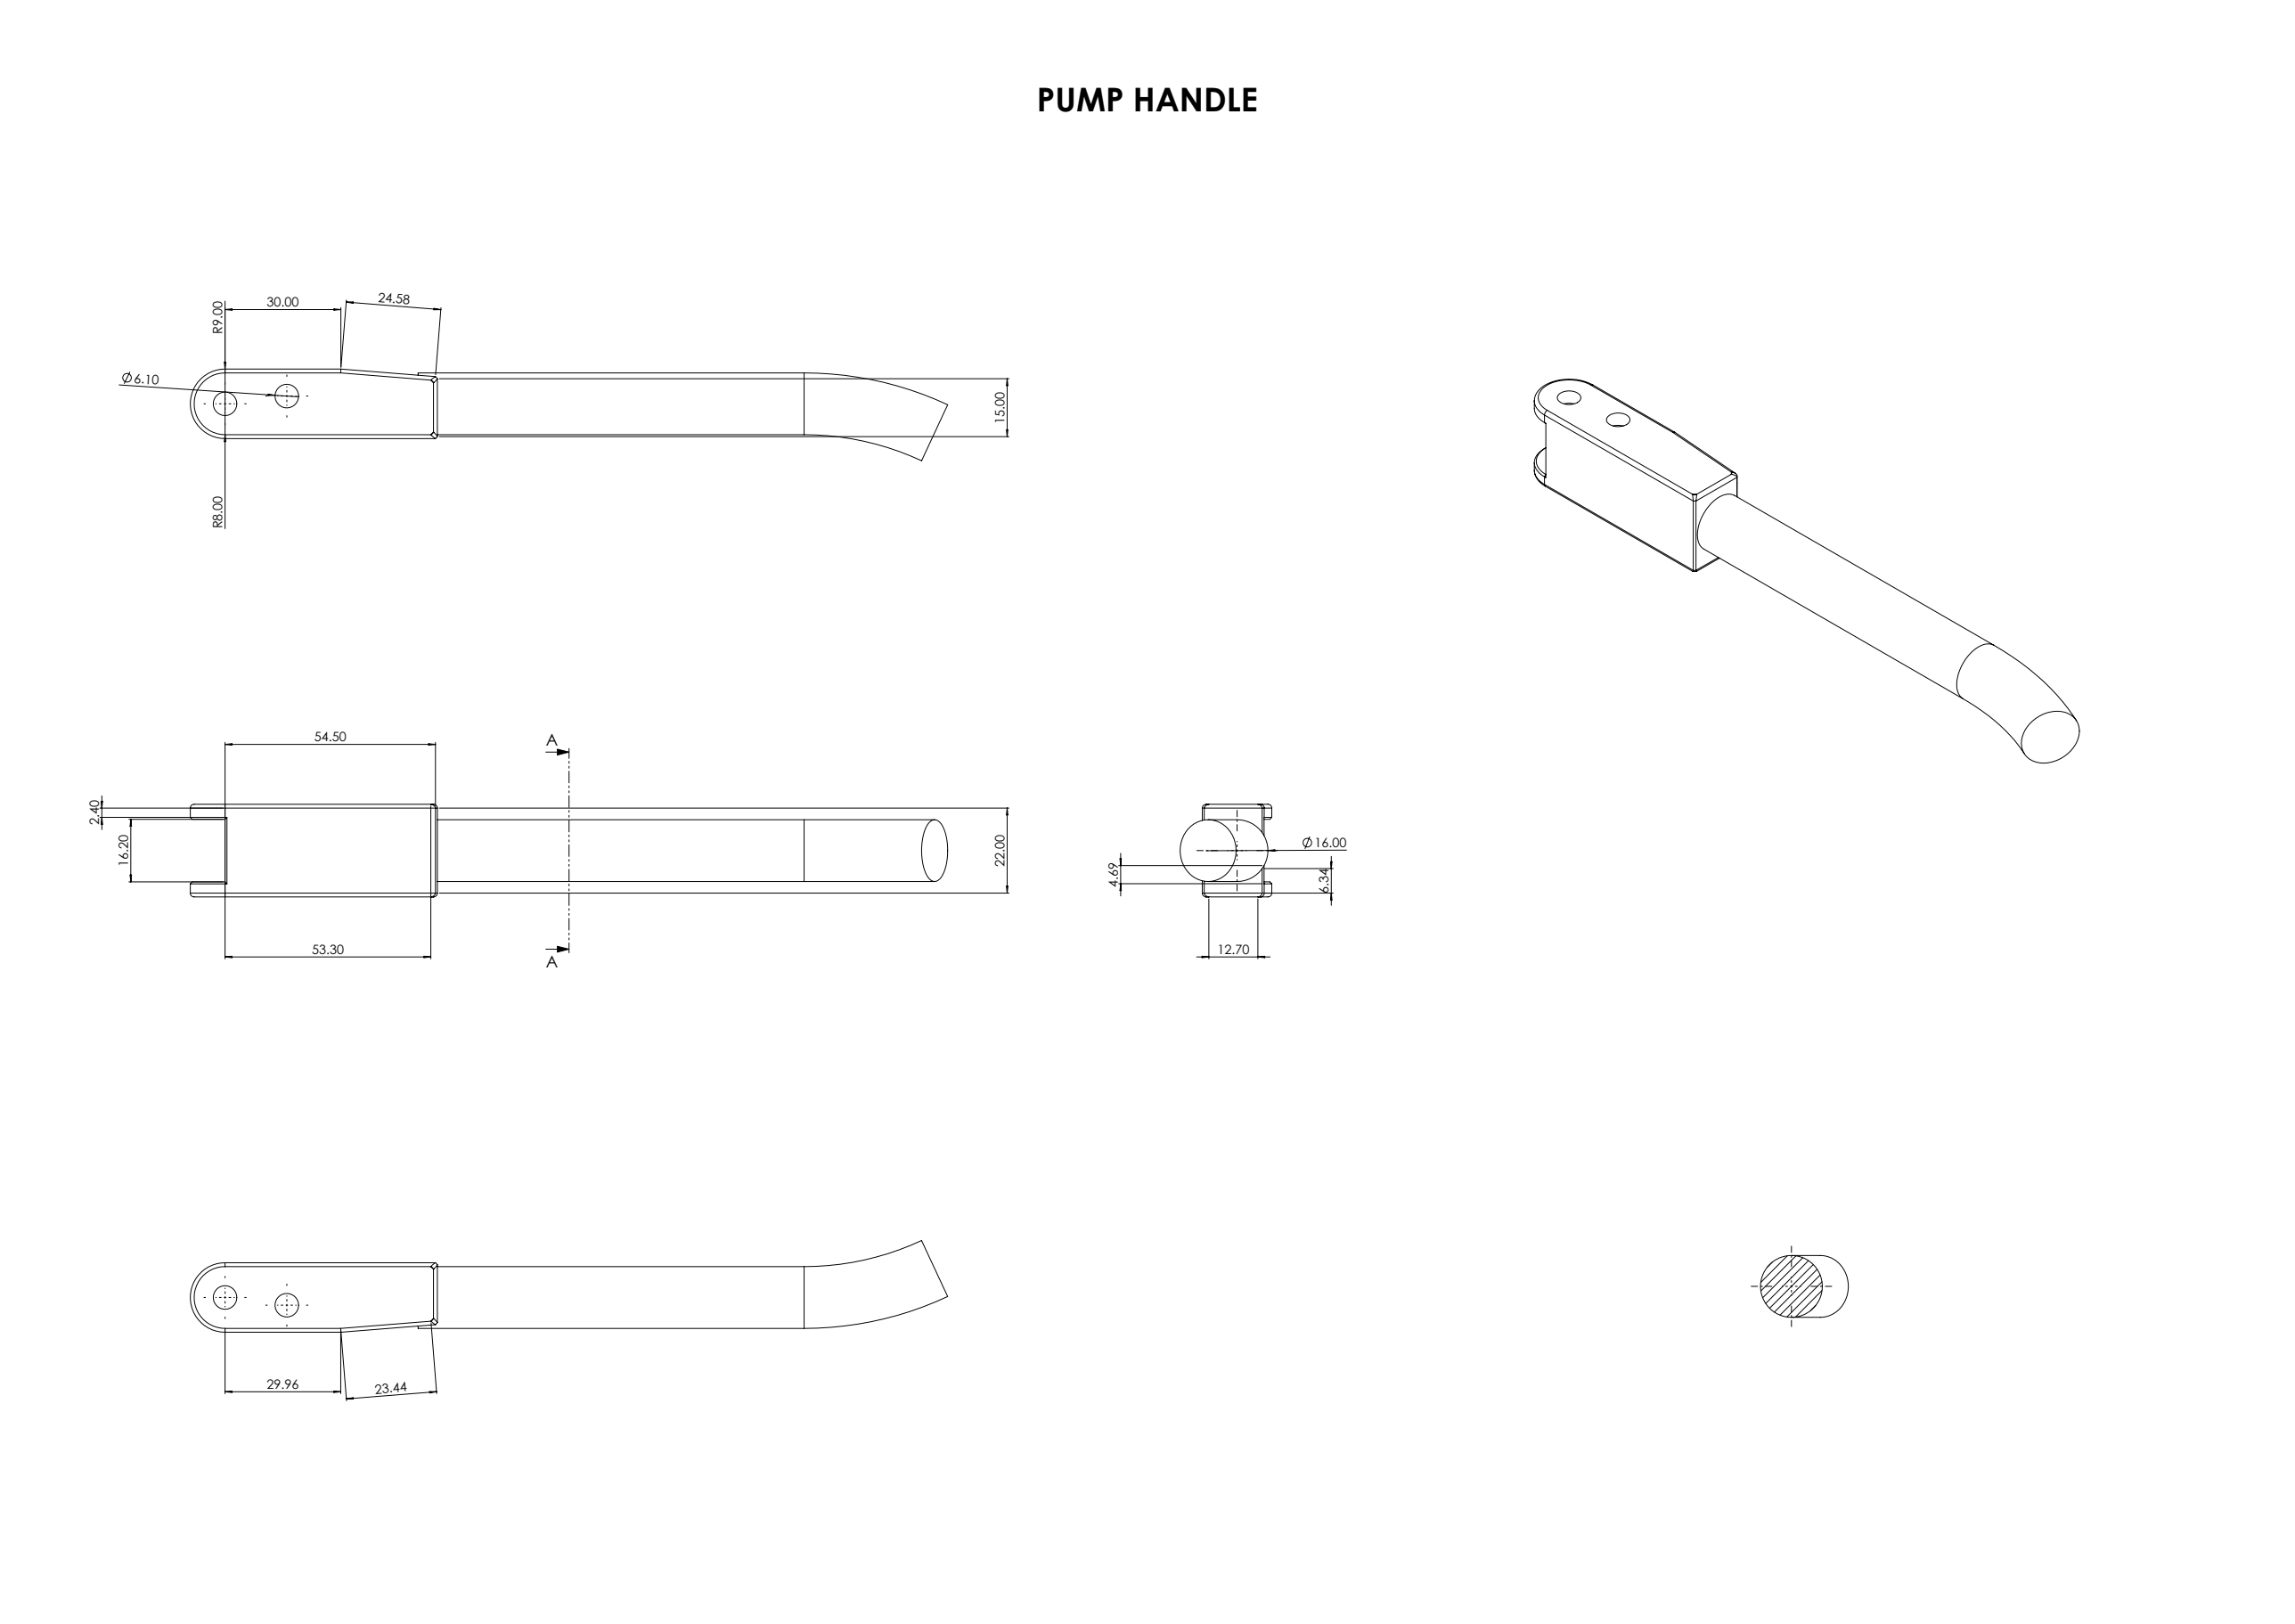
ISO-10303-21;
HEADER;
/* Generated by software containing ST-Developer
 * from STEP Tools, Inc. (www.steptools.com) 
 */

FILE_DESCRIPTION(
/* description */ (''),
/* implementation_level */ '2;1');

FILE_NAME(
/* name */ '14_Pump_Handle.step',
/* time_stamp */ '2026-10-26T03:55:20-07:00',
/* author */ (''),
/* organization */ (''),
/* preprocessor_version */ 'ST-DEVELOPER v20.2',
/* originating_system */ 'Autodesk Translation Framework v15.15.0.0',
/* authorisation */ '');

FILE_SCHEMA (('AUTOMOTIVE_DESIGN { 1 0 10303 214 3 1 1 }'));
ENDSEC;

DATA;
#10=MECHANICAL_DESIGN_GEOMETRIC_PRESENTATION_REPRESENTATION('',(#189),#45236);
#149=SHAPE_REPRESENTATION_RELATIONSHIP('SRR','None',#45328,#169);
#169=ADVANCED_BREP_SHAPE_REPRESENTATION('',(#209),#45230);
#189=STYLED_ITEM('',(#45498),#209);
#209=MANIFOLD_SOLID_BREP('Body1',#16531);
#225=TOROIDAL_SURFACE('',#17931,8.,1.);
#226=TOROIDAL_SURFACE('',#17938,8.,1.);
#227=TOROIDAL_SURFACE('',#17951,79.9999999999995,8.);
#252=ELLIPSE('',#17900,10.8879054120476,8.);
#253=ELLIPSE('',#17908,10.8879054120476,8.);
#254=ELLIPSE('',#17918,1.00079713248425,1.);
#255=ELLIPSE('',#17937,1.00079713248425,1.);
#790=B_SPLINE_CURVE_WITH_KNOTS('',3,(#44019,#44020,#44021,#44022,#44023,
#44024,#44025,#44026,#44027,#44028,#44029,#44030,#44031,#44032,#44033,#44034,
#44035,#44036,#44037,#44038,#44039,#44040,#44041,#44042,#44043,#44044,#44045,
#44046,#44047,#44048,#44049,#44050,#44051,#44052,#44053,#44054,#44055,#44056,
#44057,#44058,#44059,#44060,#44061,#44062,#44063,#44064,#44065,#44066,#44067,
#44068,#44069,#44070,#44071,#44072,#44073),.UNSPECIFIED.,.F.,.F.,(4,3,3,
3,3,3,3,3,3,3,3,3,3,3,3,3,3,3,4),(0.,0.0457286896420428,0.093735766404543,
0.144908104483403,0.201496379478659,0.273083254680907,0.346956864852629,
0.403665327235726,0.454892838429364,0.50491934325277,0.554438098871657,
0.607768246203659,0.669007112544933,0.7517553344087,0.813816500806525,0.866510270075527,
0.916070793074055,0.962308549660881,1.),.UNSPECIFIED.);
#791=B_SPLINE_CURVE_WITH_KNOTS('',3,(#44075,#44076,#44077,#44078),
 .UNSPECIFIED.,.F.,.F.,(4,4),(0.,1.),.UNSPECIFIED.);
#792=B_SPLINE_CURVE_WITH_KNOTS('',3,(#44080,#44081,#44082,#44083,#44084,
#44085,#44086,#44087,#44088,#44089,#44090,#44091,#44092,#44093,#44094,#44095,
#44096,#44097,#44098,#44099,#44100,#44101,#44102,#44103,#44104,#44105,#44106,
#44107,#44108,#44109,#44110,#44111,#44112,#44113,#44114,#44115,#44116,#44117,
#44118,#44119,#44120,#44121,#44122,#44123,#44124,#44125,#44126,#44127,#44128,
#44129,#44130,#44131,#44132,#44133,#44134),.UNSPECIFIED.,.F.,.F.,(4,3,3,
3,3,3,3,3,3,3,3,3,3,3,3,3,3,3,4),(0.,0.0457354346940703,0.0937501435458722,
0.144931624161072,0.20153359300957,0.273162634682721,0.347001992162202,
0.403710204556331,0.454939815804421,0.505015264674136,0.55453467353116,
0.607869111005662,0.669124504105853,0.75184337807939,0.813882533559542,
0.866563287605176,0.916113481178306,0.962343356347582,1.),.UNSPECIFIED.);
#793=B_SPLINE_CURVE_WITH_KNOTS('',3,(#44161,#44162,#44163,#44164,#44165,
#44166),.UNSPECIFIED.,.F.,.F.,(4,1,1,4),(-1.83137755752329,-1.04650146144188,
-0.52325073072094,-1.12036785251785E-15),.UNSPECIFIED.);
#794=B_SPLINE_CURVE_WITH_KNOTS('',3,(#44169,#44170,#44171,#44172,#44173,
#44174),.UNSPECIFIED.,.F.,.F.,(4,1,1,4),(1.12036785251785E-15,0.52325073072094,
1.04650146144188,1.83137755752329),.UNSPECIFIED.);
#795=B_SPLINE_CURVE_WITH_KNOTS('',3,(#44202,#44203,#44204,#44205,#44206,
#44207,#44208),.UNSPECIFIED.,.F.,.F.,(4,1,1,1,4),(-1.84798528578773,-1.0559915918787,
-0.527995795939349,-0.263997897969673,2.22044604925035E-15),
 .UNSPECIFIED.);
#796=B_SPLINE_CURVE_WITH_KNOTS('',3,(#44209,#44210,#44211,#44212,#44213,
#44214,#44215,#44216,#44217,#44218,#44219,#44220,#44221,#44222,#44223,#44224,
#44225,#44226,#44227,#44228,#44229,#44230,#44231,#44232,#44233,#44234,#44235,
#44236,#44237,#44238,#44239,#44240,#44241,#44242,#44243,#44244,#44245,#44246,
#44247,#44248,#44249,#44250,#44251,#44252,#44253,#44254,#44255,#44256,#44257,
#44258,#44259,#44260,#44261,#44262,#44263),.UNSPECIFIED.,.F.,.F.,(4,3,3,
3,3,3,3,3,3,3,3,3,3,3,3,3,3,3,4),(0.,0.0457132863749496,0.0937034140726246,
0.144856244328766,0.201417245857591,0.272937663581204,0.346860860114579,
0.403562222955401,0.454780120675855,0.503694405033869,0.553118113908822,
0.606292311523956,0.667190059273958,0.750392544455468,0.812794408341601,
0.865541001719504,0.91513380035021,0.961377819679936,1.),.UNSPECIFIED.);
#797=B_SPLINE_CURVE_WITH_KNOTS('',3,(#44305,#44306,#44307,#44308,#44309,
#44310,#44311,#44312,#44313,#44314,#44315,#44316,#44317,#44318,#44319,#44320,
#44321,#44322,#44323,#44324,#44325,#44326,#44327,#44328,#44329,#44330,#44331,
#44332,#44333,#44334,#44335,#44336,#44337,#44338,#44339,#44340,#44341,#44342,
#44343,#44344,#44345,#44346,#44347,#44348,#44349,#44350,#44351,#44352,#44353,
#44354,#44355,#44356,#44357,#44358,#44359),.UNSPECIFIED.,.F.,.F.,(4,3,3,
3,3,3,3,3,3,3,3,3,3,3,3,3,3,3,4),(0.,0.0457286896420497,0.0937357664051448,
0.144908104483507,0.201496379477572,0.273083254679073,0.34695686485381,
0.403665327236825,0.454892838430446,0.504919343256333,0.554438098874351,
0.607768246204756,0.669007112545538,0.751755334409154,0.813816500806865,
0.866510270075756,0.916070793073951,0.962308549660669,1.),.UNSPECIFIED.);
#798=B_SPLINE_CURVE_WITH_KNOTS('',3,(#44361,#44362,#44363,#44364),
 .UNSPECIFIED.,.F.,.F.,(4,4),(0.,1.),.UNSPECIFIED.);
#799=B_SPLINE_CURVE_WITH_KNOTS('',3,(#44366,#44367,#44368,#44369,#44370,
#44371,#44372,#44373,#44374,#44375,#44376,#44377,#44378,#44379,#44380,#44381,
#44382,#44383,#44384,#44385,#44386,#44387,#44388,#44389,#44390,#44391,#44392,
#44393,#44394,#44395,#44396,#44397,#44398,#44399,#44400,#44401,#44402,#44403,
#44404,#44405,#44406,#44407,#44408,#44409,#44410,#44411,#44412,#44413,#44414,
#44415,#44416,#44417,#44418,#44419,#44420),.UNSPECIFIED.,.F.,.F.,(4,3,3,
3,3,3,3,3,3,3,3,3,3,3,3,3,3,3,4),(0.,0.0457354346944535,0.0937501435463771,
0.144931624161605,0.201533593009091,0.273162634682324,0.347001992161254,
0.40371020455566,0.454939815803727,0.505015264672052,0.554534673528658,
0.607869111002009,0.669124504101831,0.751843378076374,0.81388253355728,
0.866563287602945,0.916113481176235,0.962343356345523,1.),.UNSPECIFIED.);
#800=B_SPLINE_CURVE_WITH_KNOTS('',3,(#44446,#44447,#44448,#44449,#44450,
#44451),.UNSPECIFIED.,.F.,.F.,(4,1,1,4),(-1.83137755752328,-1.04650146144188,
-0.523250730720938,-1.19348975147204E-15),.UNSPECIFIED.);
#801=B_SPLINE_CURVE_WITH_KNOTS('',3,(#44452,#44453,#44454,#44455,#44456,
#44457),.UNSPECIFIED.,.F.,.F.,(4,1,1,4),(1.19348975147204E-15,0.523250730720938,
1.04650146144188,1.83137755752328),.UNSPECIFIED.);
#802=B_SPLINE_CURVE_WITH_KNOTS('',3,(#44508,#44509,#44510,#44511),
 .UNSPECIFIED.,.F.,.F.,(4,4),(0.,1.),.UNSPECIFIED.);
#803=B_SPLINE_CURVE_WITH_KNOTS('',3,(#44512,#44513,#44514,#44515,#44516,
#44517,#44518,#44519,#44520,#44521,#44522,#44523,#44524,#44525,#44526,#44527,
#44528,#44529,#44530,#44531,#44532,#44533,#44534,#44535,#44536,#44537,#44538,
#44539,#44540,#44541,#44542,#44543,#44544,#44545,#44546,#44547,#44548,#44549,
#44550,#44551,#44552,#44553,#44554,#44555,#44556,#44557,#44558,#44559,#44560,
#44561,#44562,#44563,#44564,#44565,#44566),.UNSPECIFIED.,.F.,.F.,(4,3,3,
3,3,3,3,3,3,3,3,3,3,3,3,3,3,3,4),(0.,0.0457192684189794,0.0937161650457905,
0.144877103812885,0.201450247057813,0.273008005410247,0.346900713129524,
0.403601873101028,0.454821643624999,0.503755854254589,0.553178607570083,
0.606353906221449,0.667259789018953,0.750444841764215,0.812833631323161,
0.865569987859207,0.915154528460697,0.961391964978838,1.),.UNSPECIFIED.);
#804=B_SPLINE_CURVE_WITH_KNOTS('',3,(#44601,#44602,#44603,#44604,#44605,
#44606,#44607,#44608,#44609,#44610,#44611,#44612,#44613,#44614,#44615,#44616,
#44617,#44618,#44619,#44620,#44621,#44622,#44623,#44624,#44625,#44626,#44627,
#44628,#44629,#44630,#44631,#44632,#44633,#44634,#44635,#44636,#44637,#44638,
#44639,#44640,#44641,#44642,#44643,#44644,#44645,#44646,#44647,#44648,#44649,
#44650,#44651,#44652,#44653,#44654,#44655),.UNSPECIFIED.,.F.,.F.,(4,3,3,
3,3,3,3,3,3,3,3,3,3,3,3,3,3,3,4),(0.,0.0457132863751776,0.093703414073713,
0.144856244329965,0.201417245862007,0.272937663588709,0.346860860113243,
0.403562222954799,0.454780120675612,0.503694405126385,0.553118114005435,
0.60629231162977,0.667190059400792,0.750392544550594,0.812794408412946,
0.865541001786358,0.915133800413365,0.961377819741294,1.),.UNSPECIFIED.);
#805=B_SPLINE_CURVE_WITH_KNOTS('',3,(#44657,#44658,#44659,#44660),
 .UNSPECIFIED.,.F.,.F.,(4,4),(0.,1.),.UNSPECIFIED.);
#806=B_SPLINE_CURVE_WITH_KNOTS('',3,(#44662,#44663,#44664,#44665,#44666,
#44667,#44668,#44669,#44670,#44671,#44672,#44673,#44674,#44675,#44676,#44677,
#44678,#44679,#44680,#44681,#44682,#44683,#44684,#44685,#44686,#44687,#44688,
#44689,#44690,#44691,#44692,#44693,#44694,#44695,#44696,#44697,#44698,#44699,
#44700,#44701,#44702,#44703,#44704,#44705,#44706,#44707,#44708,#44709,#44710,
#44711,#44712,#44713,#44714,#44715,#44716),.UNSPECIFIED.,.F.,.F.,(4,3,3,
3,3,3,3,3,3,3,3,3,3,3,3,3,3,3,4),(0.,0.04571926841842,0.093716165045645,
0.144877103812341,0.201450247056974,0.273008005409813,0.346900713129314,
0.403601873101765,0.454821643626316,0.503755854294485,0.553178607611452,
0.606353906267959,0.667259789075755,0.750444841806816,0.812833631355112,
0.865569987889283,0.915154528488622,0.961391965006156,1.),.UNSPECIFIED.);
#807=B_SPLINE_CURVE_WITH_KNOTS('',3,(#44746,#44747,#44748,#44749,#44750,
#44751,#44752),.UNSPECIFIED.,.F.,.F.,(4,1,1,1,4),(-1.84798528578773,-1.0559915918787,
-0.527995795939349,-0.263997897969672,4.44089209850066E-15),
 .UNSPECIFIED.);
#808=B_SPLINE_CURVE_WITH_KNOTS('',3,(#44754,#44755,#44756,#44757,#44758,
#44759,#44760),.UNSPECIFIED.,.F.,.F.,(4,1,1,1,4),(-4.44089209850066E-15,
0.263997897969672,0.527995795939349,1.0559915918787,1.84798528578773),
 .UNSPECIFIED.);
#809=B_SPLINE_CURVE_WITH_KNOTS('',3,(#44791,#44792,#44793,#44794,#44795,
#44796,#44797),.UNSPECIFIED.,.F.,.F.,(4,1,1,1,4),(-2.22044604925035E-15,
0.263997897969673,0.527995795939349,1.0559915918787,1.84798528578773),
 .UNSPECIFIED.);
#931=B_SPLINE_SURFACE_WITH_KNOTS('',3,3,((#43985,#43986,#43987,#43988,#43989,
#43990,#43991,#43992),(#43993,#43994,#43995,#43996,#43997,#43998,#43999,
#44000),(#44001,#44002,#44003,#44004,#44005,#44006,#44007,#44008),(#44009,
#44010,#44011,#44012,#44013,#44014,#44015,#44016)),.UNSPECIFIED.,.F.,.F.,
 .F.,(4,4),(4,1,1,1,1,4),(0.,1.),(0.,0.142857142857143,0.428571428571429,
0.571428571428571,0.857142857142857,1.),.UNSPECIFIED.);
#932=B_SPLINE_SURFACE_WITH_KNOTS('',3,3,((#44136,#44137,#44138,#44139,#44140,
#44141),(#44142,#44143,#44144,#44145,#44146,#44147),(#44148,#44149,#44150,
#44151,#44152,#44153),(#44154,#44155,#44156,#44157,#44158,#44159)),
 .UNSPECIFIED.,.F.,.F.,.F.,(4,4),(4,1,1,4),(0.,1.),(-1.83137755752329,-1.04650146144188,
-0.52325073072094,-1.12036785251785E-15),.UNSPECIFIED.);
#933=B_SPLINE_SURFACE_WITH_KNOTS('',3,3,((#44271,#44272,#44273,#44274,#44275,
#44276,#44277,#44278),(#44279,#44280,#44281,#44282,#44283,#44284,#44285,
#44286),(#44287,#44288,#44289,#44290,#44291,#44292,#44293,#44294),(#44295,
#44296,#44297,#44298,#44299,#44300,#44301,#44302)),.UNSPECIFIED.,.F.,.F.,
 .F.,(4,4),(4,1,1,1,1,4),(0.,1.),(0.,0.142857142857143,0.428571428571429,
0.571428571428571,0.857142857142857,1.),.UNSPECIFIED.);
#934=B_SPLINE_SURFACE_WITH_KNOTS('',3,3,((#44422,#44423,#44424,#44425,#44426,
#44427),(#44428,#44429,#44430,#44431,#44432,#44433),(#44434,#44435,#44436,
#44437,#44438,#44439),(#44440,#44441,#44442,#44443,#44444,#44445)),
 .UNSPECIFIED.,.F.,.F.,.F.,(4,4),(4,1,1,4),(0.,1.),(-1.83137755752328,-1.04650146144188,
-0.523250730720938,-1.19348975147204E-15),.UNSPECIFIED.);
#935=B_SPLINE_SURFACE_WITH_KNOTS('',3,3,((#44475,#44476,#44477,#44478,#44479,
#44480,#44481,#44482),(#44483,#44484,#44485,#44486,#44487,#44488,#44489,
#44490),(#44491,#44492,#44493,#44494,#44495,#44496,#44497,#44498),(#44499,
#44500,#44501,#44502,#44503,#44504,#44505,#44506)),.UNSPECIFIED.,.F.,.F.,
 .F.,(4,4),(4,1,1,1,1,4),(0.,1.),(0.,0.142857142857143,0.428571428571429,
0.571428571428571,0.857142857142857,1.),.UNSPECIFIED.);
#936=B_SPLINE_SURFACE_WITH_KNOTS('',3,3,((#44567,#44568,#44569,#44570,#44571,
#44572,#44573,#44574),(#44575,#44576,#44577,#44578,#44579,#44580,#44581,
#44582),(#44583,#44584,#44585,#44586,#44587,#44588,#44589,#44590),(#44591,
#44592,#44593,#44594,#44595,#44596,#44597,#44598)),.UNSPECIFIED.,.F.,.F.,
 .F.,(4,4),(4,1,1,1,1,4),(0.,1.),(0.,0.142857142857143,0.428571428571429,
0.571428571428571,0.857142857142857,1.),.UNSPECIFIED.);
#937=B_SPLINE_SURFACE_WITH_KNOTS('',3,3,((#44718,#44719,#44720,#44721,#44722,
#44723,#44724),(#44725,#44726,#44727,#44728,#44729,#44730,#44731),(#44732,
#44733,#44734,#44735,#44736,#44737,#44738),(#44739,#44740,#44741,#44742,
#44743,#44744,#44745)),.UNSPECIFIED.,.F.,.F.,.F.,(4,4),(4,1,1,1,4),(0.,
1.),(-1.84798528578773,-1.0559915918787,-0.527995795939349,-0.263997897969672,
4.44089209850066E-15),.UNSPECIFIED.);
#938=B_SPLINE_SURFACE_WITH_KNOTS('',3,3,((#44763,#44764,#44765,#44766,#44767,
#44768,#44769),(#44770,#44771,#44772,#44773,#44774,#44775,#44776),(#44777,
#44778,#44779,#44780,#44781,#44782,#44783),(#44784,#44785,#44786,#44787,
#44788,#44789,#44790)),.UNSPECIFIED.,.F.,.F.,.F.,(4,4),(4,1,1,1,4),(0.,
1.),(-1.84798528578773,-1.0559915918787,-0.527995795939349,-0.263997897969673,
2.22044604925035E-15),.UNSPECIFIED.);
#1042=FACE_BOUND('',#3746,.T.);
#1043=FACE_BOUND('',#3747,.T.);
#1044=FACE_BOUND('',#3762,.T.);
#1045=FACE_BOUND('',#3763,.T.);
#1046=FACE_BOUND('',#3770,.T.);
#1047=FACE_BOUND('',#3771,.T.);
#1048=FACE_BOUND('',#3784,.T.);
#1049=FACE_BOUND('',#3785,.T.);
#1498=PLANE('',#17880);
#1499=PLANE('',#17881);
#1500=PLANE('',#17882);
#1501=PLANE('',#17883);
#1502=PLANE('',#17884);
#1503=PLANE('',#17885);
#1504=PLANE('',#17889);
#1505=PLANE('',#17890);
#1506=PLANE('',#17893);
#1507=PLANE('',#17894);
#1508=PLANE('',#17898);
#1509=PLANE('',#17899);
#1510=PLANE('',#17901);
#1511=PLANE('',#17902);
#1512=PLANE('',#17905);
#1513=PLANE('',#17906);
#1514=PLANE('',#17907);
#1515=PLANE('',#17909);
#1516=PLANE('',#17914);
#1517=PLANE('',#17919);
#1518=PLANE('',#17922);
#1519=PLANE('',#17923);
#1520=PLANE('',#17933);
#1521=PLANE('',#17942);
#1522=PLANE('',#17954);
#1523=PLANE('',#17955);
#1524=PLANE('',#17956);
#1525=PLANE('',#17957);
#1783=CYLINDRICAL_SURFACE('',#17903,9.);
#1784=CYLINDRICAL_SURFACE('',#17913,1.);
#1785=CYLINDRICAL_SURFACE('',#17917,1.);
#1786=CYLINDRICAL_SURFACE('',#17924,1.);
#1787=CYLINDRICAL_SURFACE('',#17926,1.);
#1788=CYLINDRICAL_SURFACE('',#17928,1.);
#1789=CYLINDRICAL_SURFACE('',#17929,1.);
#1790=CYLINDRICAL_SURFACE('',#17936,1.);
#1791=CYLINDRICAL_SURFACE('',#17941,1.);
#1792=CYLINDRICAL_SURFACE('',#17943,9.);
#1793=CYLINDRICAL_SURFACE('',#17944,3.05);
#1794=CYLINDRICAL_SURFACE('',#17945,3.05);
#1795=CYLINDRICAL_SURFACE('',#17946,3.05);
#1796=CYLINDRICAL_SURFACE('',#17947,3.05);
#1797=CYLINDRICAL_SURFACE('',#17948,8.);
#2660=FACE_OUTER_BOUND('',#3737,.T.);
#2661=FACE_OUTER_BOUND('',#3738,.T.);
#2662=FACE_OUTER_BOUND('',#3739,.T.);
#2663=FACE_OUTER_BOUND('',#3740,.T.);
#2664=FACE_OUTER_BOUND('',#3741,.T.);
#2665=FACE_OUTER_BOUND('',#3742,.T.);
#2666=FACE_OUTER_BOUND('',#3743,.T.);
#2667=FACE_OUTER_BOUND('',#3744,.T.);
#2668=FACE_OUTER_BOUND('',#3745,.T.);
#2669=FACE_OUTER_BOUND('',#3748,.T.);
#2670=FACE_OUTER_BOUND('',#3749,.T.);
#2671=FACE_OUTER_BOUND('',#3750,.T.);
#2672=FACE_OUTER_BOUND('',#3751,.T.);
#2673=FACE_OUTER_BOUND('',#3752,.T.);
#2674=FACE_OUTER_BOUND('',#3753,.T.);
#2675=FACE_OUTER_BOUND('',#3754,.T.);
#2676=FACE_OUTER_BOUND('',#3755,.T.);
#2677=FACE_OUTER_BOUND('',#3756,.T.);
#2678=FACE_OUTER_BOUND('',#3757,.T.);
#2679=FACE_OUTER_BOUND('',#3758,.T.);
#2680=FACE_OUTER_BOUND('',#3759,.T.);
#2681=FACE_OUTER_BOUND('',#3760,.T.);
#2682=FACE_OUTER_BOUND('',#3761,.T.);
#2683=FACE_OUTER_BOUND('',#3764,.T.);
#2684=FACE_OUTER_BOUND('',#3765,.T.);
#2685=FACE_OUTER_BOUND('',#3766,.T.);
#2686=FACE_OUTER_BOUND('',#3767,.T.);
#2687=FACE_OUTER_BOUND('',#3768,.T.);
#2688=FACE_OUTER_BOUND('',#3769,.T.);
#2689=FACE_OUTER_BOUND('',#3772,.T.);
#2690=FACE_OUTER_BOUND('',#3773,.T.);
#2691=FACE_OUTER_BOUND('',#3774,.T.);
#2692=FACE_OUTER_BOUND('',#3775,.T.);
#2693=FACE_OUTER_BOUND('',#3776,.T.);
#2694=FACE_OUTER_BOUND('',#3777,.T.);
#2695=FACE_OUTER_BOUND('',#3778,.T.);
#2696=FACE_OUTER_BOUND('',#3779,.T.);
#2697=FACE_OUTER_BOUND('',#3780,.T.);
#2698=FACE_OUTER_BOUND('',#3781,.T.);
#2699=FACE_OUTER_BOUND('',#3782,.T.);
#2700=FACE_OUTER_BOUND('',#3783,.T.);
#2701=FACE_OUTER_BOUND('',#3786,.T.);
#2702=FACE_OUTER_BOUND('',#3787,.T.);
#2703=FACE_OUTER_BOUND('',#3788,.T.);
#2704=FACE_OUTER_BOUND('',#3789,.T.);
#2705=FACE_OUTER_BOUND('',#3790,.T.);
#2706=FACE_OUTER_BOUND('',#3791,.T.);
#2707=FACE_OUTER_BOUND('',#3792,.T.);
#2708=FACE_OUTER_BOUND('',#3793,.T.);
#2709=FACE_OUTER_BOUND('',#3794,.T.);
#2710=FACE_OUTER_BOUND('',#3795,.T.);
#2711=FACE_OUTER_BOUND('',#3796,.T.);
#2712=FACE_OUTER_BOUND('',#3797,.T.);
#2713=FACE_OUTER_BOUND('',#3798,.T.);
#2714=FACE_OUTER_BOUND('',#3799,.T.);
#2715=FACE_OUTER_BOUND('',#3800,.T.);
#3737=EDGE_LOOP('',(#14926,#14927,#14928,#14929));
#3738=EDGE_LOOP('',(#14930,#14931,#14932,#14933));
#3739=EDGE_LOOP('',(#14934,#14935,#14936,#14937));
#3740=EDGE_LOOP('',(#14938,#14939,#14940,#14941));
#3741=EDGE_LOOP('',(#14942,#14943,#14944,#14945,#14946));
#3742=EDGE_LOOP('',(#14947,#14948,#14949,#14950));
#3743=EDGE_LOOP('',(#14951,#14952,#14953,#14954));
#3744=EDGE_LOOP('',(#14955,#14956,#14957));
#3745=EDGE_LOOP('',(#14958,#14959,#14960,#14961,#14962,#14963,#14964,#14965,
#14966));
#3746=EDGE_LOOP('',(#14967));
#3747=EDGE_LOOP('',(#14968));
#3748=EDGE_LOOP('',(#14969,#14970,#14971,#14972,#14973));
#3749=EDGE_LOOP('',(#14974,#14975,#14976));
#3750=EDGE_LOOP('',(#14977,#14978,#14979,#14980));
#3751=EDGE_LOOP('',(#14981,#14982,#14983,#14984));
#3752=EDGE_LOOP('',(#14985,#14986,#14987,#14988,#14989,#14990));
#3753=EDGE_LOOP('',(#14991,#14992,#14993,#14994));
#3754=EDGE_LOOP('',(#14995,#14996,#14997,#14998));
#3755=EDGE_LOOP('',(#14999,#15000,#15001,#15002));
#3756=EDGE_LOOP('',(#15003,#15004,#15005,#15006,#15007,#15008,#15009,#15010));
#3757=EDGE_LOOP('',(#15011,#15012,#15013,#15014));
#3758=EDGE_LOOP('',(#15015,#15016,#15017,#15018));
#3759=EDGE_LOOP('',(#15019,#15020,#15021,#15022));
#3760=EDGE_LOOP('',(#15023,#15024,#15025,#15026,#15027,#15028));
#3761=EDGE_LOOP('',(#15029,#15030,#15031,#15032,#15033,#15034,#15035));
#3762=EDGE_LOOP('',(#15036));
#3763=EDGE_LOOP('',(#15037));
#3764=EDGE_LOOP('',(#15038,#15039,#15040,#15041,#15042,#15043));
#3765=EDGE_LOOP('',(#15044,#15045,#15046,#15047,#15048,#15049,#15050));
#3766=EDGE_LOOP('',(#15051,#15052,#15053,#15054));
#3767=EDGE_LOOP('',(#15055,#15056,#15057,#15058));
#3768=EDGE_LOOP('',(#15059,#15060,#15061,#15062,#15063));
#3769=EDGE_LOOP('',(#15064,#15065,#15066,#15067,#15068,#15069,#15070,#15071,
#15072));
#3770=EDGE_LOOP('',(#15073));
#3771=EDGE_LOOP('',(#15074));
#3772=EDGE_LOOP('',(#15075,#15076,#15077,#15078,#15079,#15080,#15081,#15082,
#15083,#15084));
#3773=EDGE_LOOP('',(#15085,#15086,#15087,#15088));
#3774=EDGE_LOOP('',(#15089,#15090,#15091,#15092));
#3775=EDGE_LOOP('',(#15093,#15094,#15095,#15096));
#3776=EDGE_LOOP('',(#15097,#15098,#15099,#15100));
#3777=EDGE_LOOP('',(#15101,#15102,#15103,#15104));
#3778=EDGE_LOOP('',(#15105,#15106,#15107,#15108,#15109));
#3779=EDGE_LOOP('',(#15110,#15111,#15112,#15113,#15114));
#3780=EDGE_LOOP('',(#15115,#15116,#15117,#15118,#15119,#15120));
#3781=EDGE_LOOP('',(#15121,#15122,#15123,#15124));
#3782=EDGE_LOOP('',(#15125,#15126,#15127,#15128));
#3783=EDGE_LOOP('',(#15129,#15130,#15131,#15132,#15133,#15134,#15135));
#3784=EDGE_LOOP('',(#15136));
#3785=EDGE_LOOP('',(#15137));
#3786=EDGE_LOOP('',(#15138,#15139,#15140,#15141,#15142));
#3787=EDGE_LOOP('',(#15143,#15144,#15145,#15146));
#3788=EDGE_LOOP('',(#15147,#15148,#15149,#15150));
#3789=EDGE_LOOP('',(#15151,#15152,#15153,#15154));
#3790=EDGE_LOOP('',(#15155,#15156,#15157,#15158));
#3791=EDGE_LOOP('',(#15159,#15160,#15161,#15162));
#3792=EDGE_LOOP('',(#15163,#15164,#15165,#15166));
#3793=EDGE_LOOP('',(#15167,#15168,#15169,#15170));
#3794=EDGE_LOOP('',(#15171,#15172,#15173,#15174));
#3795=EDGE_LOOP('',(#15175,#15176,#15177,#15178,#15179,#15180,#15181,#15182,
#15183,#15184));
#3796=EDGE_LOOP('',(#15185,#15186,#15187,#15188));
#3797=EDGE_LOOP('',(#15189));
#3798=EDGE_LOOP('',(#15190,#15191));
#3799=EDGE_LOOP('',(#15192,#15193,#15194,#15195));
#3800=EDGE_LOOP('',(#15196,#15197,#15198,#15199));
#5032=LINE('',#43867,#6343);
#5033=LINE('',#43869,#6344);
#5034=LINE('',#43871,#6345);
#5035=LINE('',#43872,#6346);
#5036=LINE('',#43875,#6347);
#5037=LINE('',#43877,#6348);
#5038=LINE('',#43878,#6349);
#5039=LINE('',#43882,#6350);
#5040=LINE('',#43884,#6351);
#5041=LINE('',#43886,#6352);
#5042=LINE('',#43887,#6353);
#5043=LINE('',#43890,#6354);
#5044=LINE('',#43892,#6355);
#5045=LINE('',#43893,#6356);
#5046=LINE('',#43897,#6357);
#5047=LINE('',#43899,#6358);
#5048=LINE('',#43901,#6359);
#5049=LINE('',#43903,#6360);
#5050=LINE('',#43904,#6361);
#5051=LINE('',#43907,#6362);
#5052=LINE('',#43909,#6363);
#5053=LINE('',#43910,#6364);
#5054=LINE('',#43913,#6365);
#5055=LINE('',#43918,#6366);
#5056=LINE('',#43919,#6367);
#5057=LINE('',#43921,#6368);
#5058=LINE('',#43922,#6369);
#5059=LINE('',#43930,#6370);
#5060=LINE('',#43932,#6371);
#5061=LINE('',#43934,#6372);
#5062=LINE('',#43936,#6373);
#5063=LINE('',#43937,#6374);
#5064=LINE('',#43940,#6375);
#5065=LINE('',#43942,#6376);
#5066=LINE('',#43943,#6377);
#5067=LINE('',#43948,#6378);
#5068=LINE('',#43951,#6379);
#5069=LINE('',#43952,#6380);
#5070=LINE('',#43955,#6381);
#5071=LINE('',#43957,#6382);
#5072=LINE('',#43959,#6383);
#5073=LINE('',#43961,#6384);
#5074=LINE('',#43965,#6385);
#5075=LINE('',#43966,#6386);
#5076=LINE('',#43969,#6387);
#5077=LINE('',#43970,#6388);
#5078=LINE('',#43973,#6389);
#5079=LINE('',#43977,#6390);
#5080=LINE('',#43979,#6391);
#5081=LINE('',#43981,#6392);
#5082=LINE('',#43982,#6393);
#5083=LINE('',#43983,#6394);
#5084=LINE('',#44135,#6395);
#5085=LINE('',#44168,#6396);
#5086=LINE('',#44177,#6397);
#5087=LINE('',#44180,#6398);
#5088=LINE('',#44181,#6399);
#5089=LINE('',#44184,#6400);
#5090=LINE('',#44186,#6401);
#5091=LINE('',#44188,#6402);
#5092=LINE('',#44192,#6403);
#5093=LINE('',#44193,#6404);
#5094=LINE('',#44200,#6405);
#5095=LINE('',#44269,#6406);
#5096=LINE('',#44270,#6407);
#5097=LINE('',#44421,#6408);
#5098=LINE('',#44461,#6409);
#5099=LINE('',#44463,#6410);
#5100=LINE('',#44464,#6411);
#5101=LINE('',#44471,#6412);
#5102=LINE('',#44473,#6413);
#5103=LINE('',#44474,#6414);
#5104=LINE('',#44717,#6415);
#5105=LINE('',#44753,#6416);
#5106=LINE('',#44762,#6417);
#5107=LINE('',#44802,#6418);
#5108=LINE('',#44805,#6419);
#5109=LINE('',#44809,#6420);
#5110=LINE('',#44820,#6421);
#5111=LINE('',#44826,#6422);
#5112=LINE('',#44828,#6423);
#5113=LINE('',#44829,#6424);
#5114=LINE('',#44832,#6425);
#5115=LINE('',#44834,#6426);
#5116=LINE('',#44836,#6427);
#5117=LINE('',#44838,#6428);
#5118=LINE('',#44842,#6429);
#6343=VECTOR('',#21515,10.);
#6344=VECTOR('',#21516,10.);
#6345=VECTOR('',#21517,10.);
#6346=VECTOR('',#21518,10.);
#6347=VECTOR('',#21521,10.);
#6348=VECTOR('',#21522,10.);
#6349=VECTOR('',#21523,10.);
#6350=VECTOR('',#21526,10.);
#6351=VECTOR('',#21527,10.);
#6352=VECTOR('',#21528,10.);
#6353=VECTOR('',#21529,10.);
#6354=VECTOR('',#21532,10.);
#6355=VECTOR('',#21533,10.);
#6356=VECTOR('',#21534,10.);
#6357=VECTOR('',#21537,10.);
#6358=VECTOR('',#21538,10.);
#6359=VECTOR('',#21539,10.);
#6360=VECTOR('',#21540,10.);
#6361=VECTOR('',#21541,10.);
#6362=VECTOR('',#21544,10.);
#6363=VECTOR('',#21545,10.);
#6364=VECTOR('',#21546,10.);
#6365=VECTOR('',#21549,10.);
#6366=VECTOR('',#21556,10.);
#6367=VECTOR('',#21557,10.);
#6368=VECTOR('',#21560,10.);
#6369=VECTOR('',#21561,10.);
#6370=VECTOR('',#21568,10.);
#6371=VECTOR('',#21569,10.);
#6372=VECTOR('',#21570,10.);
#6373=VECTOR('',#21571,10.);
#6374=VECTOR('',#21572,10.);
#6375=VECTOR('',#21575,10.);
#6376=VECTOR('',#21576,10.);
#6377=VECTOR('',#21577,10.);
#6378=VECTOR('',#21582,10.);
#6379=VECTOR('',#21587,10.);
#6380=VECTOR('',#21588,10.);
#6381=VECTOR('',#21591,10.);
#6382=VECTOR('',#21592,10.);
#6383=VECTOR('',#21593,10.);
#6384=VECTOR('',#21594,10.);
#6385=VECTOR('',#21599,10.);
#6386=VECTOR('',#21600,10.);
#6387=VECTOR('',#21603,10.);
#6388=VECTOR('',#21604,10.);
#6389=VECTOR('',#21607,10.);
#6390=VECTOR('',#21612,10.);
#6391=VECTOR('',#21613,10.);
#6392=VECTOR('',#21614,10.);
#6393=VECTOR('',#21615,10.);
#6394=VECTOR('',#21616,10.);
#6395=VECTOR('',#21619,10.);
#6396=VECTOR('',#21620,10.);
#6397=VECTOR('',#21623,10.);
#6398=VECTOR('',#21626,10.);
#6399=VECTOR('',#21627,10.);
#6400=VECTOR('',#21630,10.);
#6401=VECTOR('',#21631,10.);
#6402=VECTOR('',#21632,10.);
#6403=VECTOR('',#21635,10.);
#6404=VECTOR('',#21636,10.);
#6405=VECTOR('',#21643,10.);
#6406=VECTOR('',#21650,10.);
#6407=VECTOR('',#21651,10.);
#6408=VECTOR('',#21652,10.);
#6409=VECTOR('',#21657,10.);
#6410=VECTOR('',#21660,10.);
#6411=VECTOR('',#21661,10.);
#6412=VECTOR('',#21668,10.);
#6413=VECTOR('',#21669,10.);
#6414=VECTOR('',#21670,10.);
#6415=VECTOR('',#21671,10.);
#6416=VECTOR('',#21672,10.);
#6417=VECTOR('',#21675,10.);
#6418=VECTOR('',#21682,10.);
#6419=VECTOR('',#21687,10.);
#6420=VECTOR('',#21692,10.);
#6421=VECTOR('',#21707,10.);
#6422=VECTOR('',#21716,10.);
#6423=VECTOR('',#21719,10.);
#6424=VECTOR('',#21720,10.);
#6425=VECTOR('',#21725,3.05);
#6426=VECTOR('',#21728,3.05);
#6427=VECTOR('',#21731,3.05);
#6428=VECTOR('',#21734,3.05);
#6429=VECTOR('',#21739,8.);
#6880=CIRCLE('',#17887,8.5);
#6881=CIRCLE('',#17888,9.);
#6882=CIRCLE('',#17891,3.05);
#6883=CIRCLE('',#17892,3.05);
#6884=CIRCLE('',#17896,9.);
#6885=CIRCLE('',#17897,8.5);
#6886=CIRCLE('',#17904,9.);
#6887=CIRCLE('',#17910,8.);
#6888=CIRCLE('',#17911,3.05);
#6889=CIRCLE('',#17912,3.05);
#6890=CIRCLE('',#17915,8.);
#6891=CIRCLE('',#17916,8.);
#6892=CIRCLE('',#17920,3.05);
#6893=CIRCLE('',#17921,3.05);
#6894=CIRCLE('',#17925,1.);
#6895=CIRCLE('',#17927,1.);
#6896=CIRCLE('',#17930,1.);
#6897=CIRCLE('',#17932,8.);
#6898=CIRCLE('',#17934,3.05);
#6899=CIRCLE('',#17935,3.05);
#6900=CIRCLE('',#17939,1.);
#6901=CIRCLE('',#17940,9.);
#6902=CIRCLE('',#17949,8.);
#6903=CIRCLE('',#17950,8.);
#6904=CIRCLE('',#17952,8.);
#6905=CIRCLE('',#17953,71.9999999999995);
#8299=VERTEX_POINT('',#43865);
#8300=VERTEX_POINT('',#43866);
#8301=VERTEX_POINT('',#43868);
#8302=VERTEX_POINT('',#43870);
#8303=VERTEX_POINT('',#43874);
#8304=VERTEX_POINT('',#43876);
#8305=VERTEX_POINT('',#43880);
#8306=VERTEX_POINT('',#43881);
#8307=VERTEX_POINT('',#43883);
#8308=VERTEX_POINT('',#43885);
#8309=VERTEX_POINT('',#43889);
#8310=VERTEX_POINT('',#43891);
#8311=VERTEX_POINT('',#43895);
#8312=VERTEX_POINT('',#43896);
#8313=VERTEX_POINT('',#43898);
#8314=VERTEX_POINT('',#43900);
#8315=VERTEX_POINT('',#43902);
#8316=VERTEX_POINT('',#43906);
#8317=VERTEX_POINT('',#43908);
#8318=VERTEX_POINT('',#43912);
#8319=VERTEX_POINT('',#43917);
#8320=VERTEX_POINT('',#43923);
#8321=VERTEX_POINT('',#43925);
#8322=VERTEX_POINT('',#43928);
#8323=VERTEX_POINT('',#43929);
#8324=VERTEX_POINT('',#43931);
#8325=VERTEX_POINT('',#43933);
#8326=VERTEX_POINT('',#43935);
#8327=VERTEX_POINT('',#43939);
#8328=VERTEX_POINT('',#43941);
#8329=VERTEX_POINT('',#43945);
#8330=VERTEX_POINT('',#43947);
#8331=VERTEX_POINT('',#43954);
#8332=VERTEX_POINT('',#43956);
#8333=VERTEX_POINT('',#43958);
#8334=VERTEX_POINT('',#43960);
#8335=VERTEX_POINT('',#43964);
#8336=VERTEX_POINT('',#43968);
#8337=VERTEX_POINT('',#43972);
#8338=VERTEX_POINT('',#43976);
#8339=VERTEX_POINT('',#43978);
#8340=VERTEX_POINT('',#43980);
#8341=VERTEX_POINT('',#44017);
#8342=VERTEX_POINT('',#44018);
#8343=VERTEX_POINT('',#44074);
#8344=VERTEX_POINT('',#44079);
#8345=VERTEX_POINT('',#44160);
#8346=VERTEX_POINT('',#44167);
#8347=VERTEX_POINT('',#44176);
#8348=VERTEX_POINT('',#44178);
#8349=VERTEX_POINT('',#44183);
#8350=VERTEX_POINT('',#44185);
#8351=VERTEX_POINT('',#44187);
#8352=VERTEX_POINT('',#44189);
#8353=VERTEX_POINT('',#44191);
#8354=VERTEX_POINT('',#44194);
#8355=VERTEX_POINT('',#44196);
#8356=VERTEX_POINT('',#44199);
#8357=VERTEX_POINT('',#44201);
#8358=VERTEX_POINT('',#44265);
#8359=VERTEX_POINT('',#44268);
#8360=VERTEX_POINT('',#44303);
#8361=VERTEX_POINT('',#44304);
#8362=VERTEX_POINT('',#44360);
#8363=VERTEX_POINT('',#44365);
#8364=VERTEX_POINT('',#44459);
#8365=VERTEX_POINT('',#44465);
#8366=VERTEX_POINT('',#44467);
#8367=VERTEX_POINT('',#44470);
#8368=VERTEX_POINT('',#44472);
#8369=VERTEX_POINT('',#44507);
#8370=VERTEX_POINT('',#44599);
#8371=VERTEX_POINT('',#44600);
#8372=VERTEX_POINT('',#44656);
#8373=VERTEX_POINT('',#44661);
#8374=VERTEX_POINT('',#44801);
#8375=VERTEX_POINT('',#44807);
#8376=VERTEX_POINT('',#44813);
#8377=VERTEX_POINT('',#44815);
#8378=VERTEX_POINT('',#44818);
#8379=VERTEX_POINT('',#44822);
#8380=VERTEX_POINT('',#44840);
#8381=VERTEX_POINT('',#44845);
#10526=EDGE_CURVE('',#8299,#8300,#5032,.F.);
#10527=EDGE_CURVE('',#8300,#8301,#5033,.T.);
#10528=EDGE_CURVE('',#8301,#8302,#5034,.F.);
#10529=EDGE_CURVE('',#8302,#8299,#5035,.T.);
#10530=EDGE_CURVE('',#8303,#8300,#5036,.T.);
#10531=EDGE_CURVE('',#8304,#8303,#5037,.T.);
#10532=EDGE_CURVE('',#8301,#8304,#5038,.T.);
#10533=EDGE_CURVE('',#8305,#8306,#5039,.F.);
#10534=EDGE_CURVE('',#8306,#8307,#5040,.T.);
#10535=EDGE_CURVE('',#8307,#8308,#5041,.F.);
#10536=EDGE_CURVE('',#8308,#8305,#5042,.T.);
#10537=EDGE_CURVE('',#8309,#8306,#5043,.T.);
#10538=EDGE_CURVE('',#8309,#8310,#5044,.T.);
#10539=EDGE_CURVE('',#8307,#8310,#5045,.T.);
#10540=EDGE_CURVE('',#8311,#8312,#5046,.T.);
#10541=EDGE_CURVE('',#8312,#8313,#5047,.F.);
#10542=EDGE_CURVE('',#8313,#8314,#5048,.T.);
#10543=EDGE_CURVE('',#8314,#8315,#5049,.T.);
#10544=EDGE_CURVE('',#8315,#8311,#5050,.T.);
#10545=EDGE_CURVE('',#8315,#8316,#5051,.T.);
#10546=EDGE_CURVE('',#8316,#8317,#5052,.T.);
#10547=EDGE_CURVE('',#8317,#8311,#5053,.T.);
#10548=EDGE_CURVE('',#8318,#8303,#5054,.T.);
#10549=EDGE_CURVE('',#8303,#8317,#6880,.T.);
#10550=EDGE_CURVE('',#8316,#8318,#6881,.T.);
#10551=EDGE_CURVE('',#8319,#8303,#5055,.F.);
#10552=EDGE_CURVE('',#8318,#8319,#5056,.T.);
#10553=EDGE_CURVE('',#8299,#8309,#5057,.T.);
#10554=EDGE_CURVE('',#8305,#8312,#5058,.T.);
#10555=EDGE_CURVE('',#8320,#8320,#6882,.T.);
#10556=EDGE_CURVE('',#8321,#8321,#6883,.T.);
#10557=EDGE_CURVE('',#8322,#8323,#5059,.T.);
#10558=EDGE_CURVE('',#8323,#8324,#5060,.T.);
#10559=EDGE_CURVE('',#8325,#8324,#5061,.T.);
#10560=EDGE_CURVE('',#8325,#8326,#5062,.T.);
#10561=EDGE_CURVE('',#8326,#8322,#5063,.T.);
#10562=EDGE_CURVE('',#8327,#8304,#5064,.T.);
#10563=EDGE_CURVE('',#8327,#8328,#5065,.T.);
#10564=EDGE_CURVE('',#8328,#8304,#5066,.T.);
#10565=EDGE_CURVE('',#8328,#8329,#6884,.T.);
#10566=EDGE_CURVE('',#8329,#8330,#5067,.T.);
#10567=EDGE_CURVE('',#8330,#8304,#6885,.T.);
#10568=EDGE_CURVE('',#8326,#8330,#5068,.T.);
#10569=EDGE_CURVE('',#8329,#8322,#5069,.T.);
#10570=EDGE_CURVE('',#8331,#8324,#5070,.T.);
#10571=EDGE_CURVE('',#8323,#8332,#5071,.T.);
#10572=EDGE_CURVE('',#8333,#8332,#5072,.T.);
#10573=EDGE_CURVE('',#8333,#8334,#5073,.T.);
#10574=EDGE_CURVE('',#8334,#8331,#252,.F.);
#10575=EDGE_CURVE('',#8322,#8335,#5074,.T.);
#10576=EDGE_CURVE('',#8332,#8335,#5075,.T.);
#10577=EDGE_CURVE('',#8329,#8336,#5076,.T.);
#10578=EDGE_CURVE('',#8335,#8336,#5077,.T.);
#10579=EDGE_CURVE('',#8328,#8337,#5078,.T.);
#10580=EDGE_CURVE('',#8336,#8337,#6886,.T.);
#10581=EDGE_CURVE('',#8318,#8338,#5079,.T.);
#10582=EDGE_CURVE('',#8339,#8338,#5080,.T.);
#10583=EDGE_CURVE('',#8340,#8339,#5081,.T.);
#10584=EDGE_CURVE('',#8337,#8340,#5082,.T.);
#10585=EDGE_CURVE('',#8319,#8327,#5083,.T.);
#10586=EDGE_CURVE('',#8341,#8342,#790,.T.);
#10587=EDGE_CURVE('',#8343,#8342,#791,.T.);
#10588=EDGE_CURVE('',#8343,#8344,#792,.T.);
#10589=EDGE_CURVE('',#8344,#8341,#5084,.T.);
#10590=EDGE_CURVE('',#8342,#8345,#793,.T.);
#10591=EDGE_CURVE('',#8345,#8346,#5085,.T.);
#10592=EDGE_CURVE('',#8346,#8343,#794,.T.);
#10593=EDGE_CURVE('',#8313,#8347,#5086,.T.);
#10594=EDGE_CURVE('',#8348,#8347,#253,.T.);
#10595=EDGE_CURVE('',#8348,#8346,#5087,.T.);
#10596=EDGE_CURVE('',#8345,#8314,#5088,.T.);
#10597=EDGE_CURVE('',#8349,#8344,#5089,.T.);
#10598=EDGE_CURVE('',#8350,#8349,#5090,.T.);
#10599=EDGE_CURVE('',#8351,#8350,#5091,.T.);
#10600=EDGE_CURVE('',#8352,#8351,#6887,.T.);
#10601=EDGE_CURVE('',#8353,#8352,#5092,.T.);
#10602=EDGE_CURVE('',#8341,#8353,#5093,.T.);
#10603=EDGE_CURVE('',#8354,#8354,#6888,.T.);
#10604=EDGE_CURVE('',#8355,#8355,#6889,.T.);
#10605=EDGE_CURVE('',#8346,#8356,#5094,.T.);
#10606=EDGE_CURVE('',#8357,#8356,#795,.T.);
#10607=EDGE_CURVE('',#8349,#8357,#796,.T.);
#10608=EDGE_CURVE('',#8348,#8358,#6890,.T.);
#10609=EDGE_CURVE('',#8358,#8334,#6891,.T.);
#10610=EDGE_CURVE('',#8359,#8333,#5095,.T.);
#10611=EDGE_CURVE('',#8356,#8359,#5096,.T.);
#10612=EDGE_CURVE('',#8360,#8361,#797,.T.);
#10613=EDGE_CURVE('',#8362,#8361,#798,.T.);
#10614=EDGE_CURVE('',#8362,#8363,#799,.T.);
#10615=EDGE_CURVE('',#8363,#8360,#5097,.T.);
#10616=EDGE_CURVE('',#8361,#8333,#800,.T.);
#10617=EDGE_CURVE('',#8332,#8362,#801,.T.);
#10618=EDGE_CURVE('',#8364,#8335,#254,.T.);
#10619=EDGE_CURVE('',#8364,#8363,#5098,.T.);
#10620=EDGE_CURVE('',#8325,#8308,#5099,.T.);
#10621=EDGE_CURVE('',#8310,#8302,#5100,.T.);
#10622=EDGE_CURVE('',#8365,#8365,#6892,.T.);
#10623=EDGE_CURVE('',#8366,#8366,#6893,.T.);
#10624=EDGE_CURVE('',#8331,#8367,#5101,.T.);
#10625=EDGE_CURVE('',#8367,#8368,#5102,.T.);
#10626=EDGE_CURVE('',#8368,#8347,#5103,.T.);
#10627=EDGE_CURVE('',#8369,#8357,#802,.T.);
#10628=EDGE_CURVE('',#8369,#8350,#803,.T.);
#10629=EDGE_CURVE('',#8370,#8371,#804,.T.);
#10630=EDGE_CURVE('',#8372,#8371,#805,.T.);
#10631=EDGE_CURVE('',#8372,#8373,#806,.T.);
#10632=EDGE_CURVE('',#8373,#8370,#5104,.T.);
#10633=EDGE_CURVE('',#8371,#8340,#807,.T.);
#10634=EDGE_CURVE('',#8340,#8359,#5105,.T.);
#10635=EDGE_CURVE('',#8359,#8372,#808,.T.);
#10636=EDGE_CURVE('',#8339,#8356,#5106,.T.);
#10637=EDGE_CURVE('',#8339,#8369,#809,.T.);
#10638=EDGE_CURVE('',#8338,#8351,#6894,.T.);
#10639=EDGE_CURVE('',#8370,#8374,#5107,.T.);
#10640=EDGE_CURVE('',#8337,#8374,#6895,.T.);
#10641=EDGE_CURVE('',#8360,#8373,#5108,.T.);
#10642=EDGE_CURVE('',#8336,#8375,#6896,.T.);
#10643=EDGE_CURVE('',#8375,#8364,#5109,.T.);
#10644=EDGE_CURVE('',#8374,#8375,#6897,.T.);
#10645=EDGE_CURVE('',#8376,#8376,#6898,.T.);
#10646=EDGE_CURVE('',#8377,#8377,#6899,.T.);
#10647=EDGE_CURVE('',#8353,#8378,#255,.T.);
#10648=EDGE_CURVE('',#8378,#8345,#5110,.T.);
#10649=EDGE_CURVE('',#8379,#8352,#6900,.T.);
#10650=EDGE_CURVE('',#8338,#8379,#6901,.T.);
#10651=EDGE_CURVE('',#8379,#8378,#5111,.T.);
#10652=EDGE_CURVE('',#8315,#8378,#5112,.T.);
#10653=EDGE_CURVE('',#8316,#8379,#5113,.T.);
#10654=EDGE_CURVE('',#8366,#8377,#5114,.T.);
#10655=EDGE_CURVE('',#8355,#8321,#5115,.T.);
#10656=EDGE_CURVE('',#8365,#8376,#5116,.T.);
#10657=EDGE_CURVE('',#8354,#8320,#5117,.T.);
#10658=EDGE_CURVE('',#8380,#8380,#6902,.T.);
#10659=EDGE_CURVE('',#8380,#8358,#5118,.T.);
#10660=EDGE_CURVE('',#8368,#8367,#6903,.T.);
#10661=EDGE_CURVE('',#8381,#8381,#6904,.T.);
#10662=EDGE_CURVE('',#8381,#8380,#6905,.T.);
#14926=ORIENTED_EDGE('',*,*,#10526,.T.);
#14927=ORIENTED_EDGE('',*,*,#10527,.T.);
#14928=ORIENTED_EDGE('',*,*,#10528,.T.);
#14929=ORIENTED_EDGE('',*,*,#10529,.T.);
#14930=ORIENTED_EDGE('',*,*,#10527,.F.);
#14931=ORIENTED_EDGE('',*,*,#10530,.F.);
#14932=ORIENTED_EDGE('',*,*,#10531,.F.);
#14933=ORIENTED_EDGE('',*,*,#10532,.F.);
#14934=ORIENTED_EDGE('',*,*,#10533,.T.);
#14935=ORIENTED_EDGE('',*,*,#10534,.T.);
#14936=ORIENTED_EDGE('',*,*,#10535,.T.);
#14937=ORIENTED_EDGE('',*,*,#10536,.T.);
#14938=ORIENTED_EDGE('',*,*,#10534,.F.);
#14939=ORIENTED_EDGE('',*,*,#10537,.F.);
#14940=ORIENTED_EDGE('',*,*,#10538,.T.);
#14941=ORIENTED_EDGE('',*,*,#10539,.F.);
#14942=ORIENTED_EDGE('',*,*,#10540,.T.);
#14943=ORIENTED_EDGE('',*,*,#10541,.T.);
#14944=ORIENTED_EDGE('',*,*,#10542,.T.);
#14945=ORIENTED_EDGE('',*,*,#10543,.T.);
#14946=ORIENTED_EDGE('',*,*,#10544,.T.);
#14947=ORIENTED_EDGE('',*,*,#10545,.T.);
#14948=ORIENTED_EDGE('',*,*,#10546,.T.);
#14949=ORIENTED_EDGE('',*,*,#10547,.T.);
#14950=ORIENTED_EDGE('',*,*,#10544,.F.);
#14951=ORIENTED_EDGE('',*,*,#10548,.T.);
#14952=ORIENTED_EDGE('',*,*,#10549,.T.);
#14953=ORIENTED_EDGE('',*,*,#10546,.F.);
#14954=ORIENTED_EDGE('',*,*,#10550,.T.);
#14955=ORIENTED_EDGE('',*,*,#10551,.T.);
#14956=ORIENTED_EDGE('',*,*,#10548,.F.);
#14957=ORIENTED_EDGE('',*,*,#10552,.T.);
#14958=ORIENTED_EDGE('',*,*,#10540,.F.);
#14959=ORIENTED_EDGE('',*,*,#10547,.F.);
#14960=ORIENTED_EDGE('',*,*,#10549,.F.);
#14961=ORIENTED_EDGE('',*,*,#10530,.T.);
#14962=ORIENTED_EDGE('',*,*,#10526,.F.);
#14963=ORIENTED_EDGE('',*,*,#10553,.T.);
#14964=ORIENTED_EDGE('',*,*,#10537,.T.);
#14965=ORIENTED_EDGE('',*,*,#10533,.F.);
#14966=ORIENTED_EDGE('',*,*,#10554,.T.);
#14967=ORIENTED_EDGE('',*,*,#10555,.T.);
#14968=ORIENTED_EDGE('',*,*,#10556,.T.);
#14969=ORIENTED_EDGE('',*,*,#10557,.T.);
#14970=ORIENTED_EDGE('',*,*,#10558,.T.);
#14971=ORIENTED_EDGE('',*,*,#10559,.F.);
#14972=ORIENTED_EDGE('',*,*,#10560,.T.);
#14973=ORIENTED_EDGE('',*,*,#10561,.T.);
#14974=ORIENTED_EDGE('',*,*,#10562,.F.);
#14975=ORIENTED_EDGE('',*,*,#10563,.T.);
#14976=ORIENTED_EDGE('',*,*,#10564,.T.);
#14977=ORIENTED_EDGE('',*,*,#10564,.F.);
#14978=ORIENTED_EDGE('',*,*,#10565,.T.);
#14979=ORIENTED_EDGE('',*,*,#10566,.T.);
#14980=ORIENTED_EDGE('',*,*,#10567,.T.);
#14981=ORIENTED_EDGE('',*,*,#10568,.T.);
#14982=ORIENTED_EDGE('',*,*,#10566,.F.);
#14983=ORIENTED_EDGE('',*,*,#10569,.T.);
#14984=ORIENTED_EDGE('',*,*,#10561,.F.);
#14985=ORIENTED_EDGE('',*,*,#10570,.T.);
#14986=ORIENTED_EDGE('',*,*,#10558,.F.);
#14987=ORIENTED_EDGE('',*,*,#10571,.T.);
#14988=ORIENTED_EDGE('',*,*,#10572,.F.);
#14989=ORIENTED_EDGE('',*,*,#10573,.T.);
#14990=ORIENTED_EDGE('',*,*,#10574,.T.);
#14991=ORIENTED_EDGE('',*,*,#10557,.F.);
#14992=ORIENTED_EDGE('',*,*,#10575,.T.);
#14993=ORIENTED_EDGE('',*,*,#10576,.F.);
#14994=ORIENTED_EDGE('',*,*,#10571,.F.);
#14995=ORIENTED_EDGE('',*,*,#10569,.F.);
#14996=ORIENTED_EDGE('',*,*,#10577,.T.);
#14997=ORIENTED_EDGE('',*,*,#10578,.F.);
#14998=ORIENTED_EDGE('',*,*,#10575,.F.);
#14999=ORIENTED_EDGE('',*,*,#10565,.F.);
#15000=ORIENTED_EDGE('',*,*,#10579,.T.);
#15001=ORIENTED_EDGE('',*,*,#10580,.F.);
#15002=ORIENTED_EDGE('',*,*,#10577,.F.);
#15003=ORIENTED_EDGE('',*,*,#10552,.F.);
#15004=ORIENTED_EDGE('',*,*,#10581,.T.);
#15005=ORIENTED_EDGE('',*,*,#10582,.F.);
#15006=ORIENTED_EDGE('',*,*,#10583,.F.);
#15007=ORIENTED_EDGE('',*,*,#10584,.F.);
#15008=ORIENTED_EDGE('',*,*,#10579,.F.);
#15009=ORIENTED_EDGE('',*,*,#10563,.F.);
#15010=ORIENTED_EDGE('',*,*,#10585,.F.);
#15011=ORIENTED_EDGE('',*,*,#10531,.T.);
#15012=ORIENTED_EDGE('',*,*,#10551,.F.);
#15013=ORIENTED_EDGE('',*,*,#10585,.T.);
#15014=ORIENTED_EDGE('',*,*,#10562,.T.);
#15015=ORIENTED_EDGE('',*,*,#10586,.T.);
#15016=ORIENTED_EDGE('',*,*,#10587,.F.);
#15017=ORIENTED_EDGE('',*,*,#10588,.T.);
#15018=ORIENTED_EDGE('',*,*,#10589,.T.);
#15019=ORIENTED_EDGE('',*,*,#10587,.T.);
#15020=ORIENTED_EDGE('',*,*,#10590,.T.);
#15021=ORIENTED_EDGE('',*,*,#10591,.T.);
#15022=ORIENTED_EDGE('',*,*,#10592,.T.);
#15023=ORIENTED_EDGE('',*,*,#10593,.T.);
#15024=ORIENTED_EDGE('',*,*,#10594,.F.);
#15025=ORIENTED_EDGE('',*,*,#10595,.T.);
#15026=ORIENTED_EDGE('',*,*,#10591,.F.);
#15027=ORIENTED_EDGE('',*,*,#10596,.T.);
#15028=ORIENTED_EDGE('',*,*,#10542,.F.);
#15029=ORIENTED_EDGE('',*,*,#10589,.F.);
#15030=ORIENTED_EDGE('',*,*,#10597,.F.);
#15031=ORIENTED_EDGE('',*,*,#10598,.F.);
#15032=ORIENTED_EDGE('',*,*,#10599,.F.);
#15033=ORIENTED_EDGE('',*,*,#10600,.F.);
#15034=ORIENTED_EDGE('',*,*,#10601,.F.);
#15035=ORIENTED_EDGE('',*,*,#10602,.F.);
#15036=ORIENTED_EDGE('',*,*,#10603,.T.);
#15037=ORIENTED_EDGE('',*,*,#10604,.T.);
#15038=ORIENTED_EDGE('',*,*,#10588,.F.);
#15039=ORIENTED_EDGE('',*,*,#10592,.F.);
#15040=ORIENTED_EDGE('',*,*,#10605,.T.);
#15041=ORIENTED_EDGE('',*,*,#10606,.F.);
#15042=ORIENTED_EDGE('',*,*,#10607,.F.);
#15043=ORIENTED_EDGE('',*,*,#10597,.T.);
#15044=ORIENTED_EDGE('',*,*,#10595,.F.);
#15045=ORIENTED_EDGE('',*,*,#10608,.T.);
#15046=ORIENTED_EDGE('',*,*,#10609,.T.);
#15047=ORIENTED_EDGE('',*,*,#10573,.F.);
#15048=ORIENTED_EDGE('',*,*,#10610,.F.);
#15049=ORIENTED_EDGE('',*,*,#10611,.F.);
#15050=ORIENTED_EDGE('',*,*,#10605,.F.);
#15051=ORIENTED_EDGE('',*,*,#10612,.T.);
#15052=ORIENTED_EDGE('',*,*,#10613,.F.);
#15053=ORIENTED_EDGE('',*,*,#10614,.T.);
#15054=ORIENTED_EDGE('',*,*,#10615,.T.);
#15055=ORIENTED_EDGE('',*,*,#10613,.T.);
#15056=ORIENTED_EDGE('',*,*,#10616,.T.);
#15057=ORIENTED_EDGE('',*,*,#10572,.T.);
#15058=ORIENTED_EDGE('',*,*,#10617,.T.);
#15059=ORIENTED_EDGE('',*,*,#10614,.F.);
#15060=ORIENTED_EDGE('',*,*,#10617,.F.);
#15061=ORIENTED_EDGE('',*,*,#10576,.T.);
#15062=ORIENTED_EDGE('',*,*,#10618,.F.);
#15063=ORIENTED_EDGE('',*,*,#10619,.T.);
#15064=ORIENTED_EDGE('',*,*,#10560,.F.);
#15065=ORIENTED_EDGE('',*,*,#10620,.T.);
#15066=ORIENTED_EDGE('',*,*,#10535,.F.);
#15067=ORIENTED_EDGE('',*,*,#10539,.T.);
#15068=ORIENTED_EDGE('',*,*,#10621,.T.);
#15069=ORIENTED_EDGE('',*,*,#10528,.F.);
#15070=ORIENTED_EDGE('',*,*,#10532,.T.);
#15071=ORIENTED_EDGE('',*,*,#10567,.F.);
#15072=ORIENTED_EDGE('',*,*,#10568,.F.);
#15073=ORIENTED_EDGE('',*,*,#10622,.T.);
#15074=ORIENTED_EDGE('',*,*,#10623,.T.);
#15075=ORIENTED_EDGE('',*,*,#10536,.F.);
#15076=ORIENTED_EDGE('',*,*,#10620,.F.);
#15077=ORIENTED_EDGE('',*,*,#10559,.T.);
#15078=ORIENTED_EDGE('',*,*,#10570,.F.);
#15079=ORIENTED_EDGE('',*,*,#10624,.T.);
#15080=ORIENTED_EDGE('',*,*,#10625,.T.);
#15081=ORIENTED_EDGE('',*,*,#10626,.T.);
#15082=ORIENTED_EDGE('',*,*,#10593,.F.);
#15083=ORIENTED_EDGE('',*,*,#10541,.F.);
#15084=ORIENTED_EDGE('',*,*,#10554,.F.);
#15085=ORIENTED_EDGE('',*,*,#10607,.T.);
#15086=ORIENTED_EDGE('',*,*,#10627,.F.);
#15087=ORIENTED_EDGE('',*,*,#10628,.T.);
#15088=ORIENTED_EDGE('',*,*,#10598,.T.);
#15089=ORIENTED_EDGE('',*,*,#10629,.T.);
#15090=ORIENTED_EDGE('',*,*,#10630,.F.);
#15091=ORIENTED_EDGE('',*,*,#10631,.T.);
#15092=ORIENTED_EDGE('',*,*,#10632,.T.);
#15093=ORIENTED_EDGE('',*,*,#10630,.T.);
#15094=ORIENTED_EDGE('',*,*,#10633,.T.);
#15095=ORIENTED_EDGE('',*,*,#10634,.T.);
#15096=ORIENTED_EDGE('',*,*,#10635,.T.);
#15097=ORIENTED_EDGE('',*,*,#10634,.F.);
#15098=ORIENTED_EDGE('',*,*,#10583,.T.);
#15099=ORIENTED_EDGE('',*,*,#10636,.T.);
#15100=ORIENTED_EDGE('',*,*,#10611,.T.);
#15101=ORIENTED_EDGE('',*,*,#10627,.T.);
#15102=ORIENTED_EDGE('',*,*,#10606,.T.);
#15103=ORIENTED_EDGE('',*,*,#10636,.F.);
#15104=ORIENTED_EDGE('',*,*,#10637,.T.);
#15105=ORIENTED_EDGE('',*,*,#10628,.F.);
#15106=ORIENTED_EDGE('',*,*,#10637,.F.);
#15107=ORIENTED_EDGE('',*,*,#10582,.T.);
#15108=ORIENTED_EDGE('',*,*,#10638,.T.);
#15109=ORIENTED_EDGE('',*,*,#10599,.T.);
#15110=ORIENTED_EDGE('',*,*,#10633,.F.);
#15111=ORIENTED_EDGE('',*,*,#10629,.F.);
#15112=ORIENTED_EDGE('',*,*,#10639,.T.);
#15113=ORIENTED_EDGE('',*,*,#10640,.F.);
#15114=ORIENTED_EDGE('',*,*,#10584,.T.);
#15115=ORIENTED_EDGE('',*,*,#10612,.F.);
#15116=ORIENTED_EDGE('',*,*,#10641,.T.);
#15117=ORIENTED_EDGE('',*,*,#10631,.F.);
#15118=ORIENTED_EDGE('',*,*,#10635,.F.);
#15119=ORIENTED_EDGE('',*,*,#10610,.T.);
#15120=ORIENTED_EDGE('',*,*,#10616,.F.);
#15121=ORIENTED_EDGE('',*,*,#10578,.T.);
#15122=ORIENTED_EDGE('',*,*,#10642,.T.);
#15123=ORIENTED_EDGE('',*,*,#10643,.T.);
#15124=ORIENTED_EDGE('',*,*,#10618,.T.);
#15125=ORIENTED_EDGE('',*,*,#10640,.T.);
#15126=ORIENTED_EDGE('',*,*,#10644,.T.);
#15127=ORIENTED_EDGE('',*,*,#10642,.F.);
#15128=ORIENTED_EDGE('',*,*,#10580,.T.);
#15129=ORIENTED_EDGE('',*,*,#10615,.F.);
#15130=ORIENTED_EDGE('',*,*,#10619,.F.);
#15131=ORIENTED_EDGE('',*,*,#10643,.F.);
#15132=ORIENTED_EDGE('',*,*,#10644,.F.);
#15133=ORIENTED_EDGE('',*,*,#10639,.F.);
#15134=ORIENTED_EDGE('',*,*,#10632,.F.);
#15135=ORIENTED_EDGE('',*,*,#10641,.F.);
#15136=ORIENTED_EDGE('',*,*,#10645,.T.);
#15137=ORIENTED_EDGE('',*,*,#10646,.T.);
#15138=ORIENTED_EDGE('',*,*,#10586,.F.);
#15139=ORIENTED_EDGE('',*,*,#10602,.T.);
#15140=ORIENTED_EDGE('',*,*,#10647,.T.);
#15141=ORIENTED_EDGE('',*,*,#10648,.T.);
#15142=ORIENTED_EDGE('',*,*,#10590,.F.);
#15143=ORIENTED_EDGE('',*,*,#10649,.T.);
#15144=ORIENTED_EDGE('',*,*,#10600,.T.);
#15145=ORIENTED_EDGE('',*,*,#10638,.F.);
#15146=ORIENTED_EDGE('',*,*,#10650,.T.);
#15147=ORIENTED_EDGE('',*,*,#10601,.T.);
#15148=ORIENTED_EDGE('',*,*,#10649,.F.);
#15149=ORIENTED_EDGE('',*,*,#10651,.T.);
#15150=ORIENTED_EDGE('',*,*,#10647,.F.);
#15151=ORIENTED_EDGE('',*,*,#10545,.F.);
#15152=ORIENTED_EDGE('',*,*,#10652,.T.);
#15153=ORIENTED_EDGE('',*,*,#10651,.F.);
#15154=ORIENTED_EDGE('',*,*,#10653,.F.);
#15155=ORIENTED_EDGE('',*,*,#10550,.F.);
#15156=ORIENTED_EDGE('',*,*,#10653,.T.);
#15157=ORIENTED_EDGE('',*,*,#10650,.F.);
#15158=ORIENTED_EDGE('',*,*,#10581,.F.);
#15159=ORIENTED_EDGE('',*,*,#10623,.F.);
#15160=ORIENTED_EDGE('',*,*,#10654,.T.);
#15161=ORIENTED_EDGE('',*,*,#10646,.F.);
#15162=ORIENTED_EDGE('',*,*,#10654,.F.);
#15163=ORIENTED_EDGE('',*,*,#10604,.F.);
#15164=ORIENTED_EDGE('',*,*,#10655,.T.);
#15165=ORIENTED_EDGE('',*,*,#10556,.F.);
#15166=ORIENTED_EDGE('',*,*,#10655,.F.);
#15167=ORIENTED_EDGE('',*,*,#10622,.F.);
#15168=ORIENTED_EDGE('',*,*,#10656,.T.);
#15169=ORIENTED_EDGE('',*,*,#10645,.F.);
#15170=ORIENTED_EDGE('',*,*,#10656,.F.);
#15171=ORIENTED_EDGE('',*,*,#10603,.F.);
#15172=ORIENTED_EDGE('',*,*,#10657,.T.);
#15173=ORIENTED_EDGE('',*,*,#10555,.F.);
#15174=ORIENTED_EDGE('',*,*,#10657,.F.);
#15175=ORIENTED_EDGE('',*,*,#10658,.F.);
#15176=ORIENTED_EDGE('',*,*,#10659,.T.);
#15177=ORIENTED_EDGE('',*,*,#10608,.F.);
#15178=ORIENTED_EDGE('',*,*,#10594,.T.);
#15179=ORIENTED_EDGE('',*,*,#10626,.F.);
#15180=ORIENTED_EDGE('',*,*,#10660,.T.);
#15181=ORIENTED_EDGE('',*,*,#10624,.F.);
#15182=ORIENTED_EDGE('',*,*,#10574,.F.);
#15183=ORIENTED_EDGE('',*,*,#10609,.F.);
#15184=ORIENTED_EDGE('',*,*,#10659,.F.);
#15185=ORIENTED_EDGE('',*,*,#10661,.F.);
#15186=ORIENTED_EDGE('',*,*,#10662,.T.);
#15187=ORIENTED_EDGE('',*,*,#10658,.T.);
#15188=ORIENTED_EDGE('',*,*,#10662,.F.);
#15189=ORIENTED_EDGE('',*,*,#10661,.T.);
#15190=ORIENTED_EDGE('',*,*,#10625,.F.);
#15191=ORIENTED_EDGE('',*,*,#10660,.F.);
#15192=ORIENTED_EDGE('',*,*,#10529,.F.);
#15193=ORIENTED_EDGE('',*,*,#10621,.F.);
#15194=ORIENTED_EDGE('',*,*,#10538,.F.);
#15195=ORIENTED_EDGE('',*,*,#10553,.F.);
#15196=ORIENTED_EDGE('',*,*,#10543,.F.);
#15197=ORIENTED_EDGE('',*,*,#10596,.F.);
#15198=ORIENTED_EDGE('',*,*,#10648,.F.);
#15199=ORIENTED_EDGE('',*,*,#10652,.F.);
#15525=CONICAL_SURFACE('',#17886,8.75,0.785398163397448);
#15526=CONICAL_SURFACE('',#17895,8.75,0.785398163397448);
#16388=ADVANCED_FACE('',(#2660),#1498,.T.);
#16389=ADVANCED_FACE('',(#2661),#1499,.T.);
#16390=ADVANCED_FACE('',(#2662),#1500,.T.);
#16391=ADVANCED_FACE('',(#2663),#1501,.T.);
#16392=ADVANCED_FACE('',(#2664),#1502,.T.);
#16393=ADVANCED_FACE('',(#2665),#1503,.T.);
#16394=ADVANCED_FACE('',(#2666),#15525,.T.);
#16395=ADVANCED_FACE('',(#2667),#1504,.T.);
#16396=ADVANCED_FACE('',(#2668,#1042,#1043),#1505,.T.);
#16397=ADVANCED_FACE('',(#2669),#1506,.T.);
#16398=ADVANCED_FACE('',(#2670),#1507,.T.);
#16399=ADVANCED_FACE('',(#2671),#15526,.T.);
#16400=ADVANCED_FACE('',(#2672),#1508,.T.);
#16401=ADVANCED_FACE('',(#2673),#1509,.T.);
#16402=ADVANCED_FACE('',(#2674),#1510,.T.);
#16403=ADVANCED_FACE('',(#2675),#1511,.T.);
#16404=ADVANCED_FACE('',(#2676),#1783,.T.);
#16405=ADVANCED_FACE('',(#2677),#1512,.T.);
#16406=ADVANCED_FACE('',(#2678),#1513,.T.);
#16407=ADVANCED_FACE('',(#2679),#931,.T.);
#16408=ADVANCED_FACE('',(#2680),#932,.T.);
#16409=ADVANCED_FACE('',(#2681),#1514,.T.);
#16410=ADVANCED_FACE('',(#2682,#1044,#1045),#1515,.F.);
#16411=ADVANCED_FACE('',(#2683),#1784,.T.);
#16412=ADVANCED_FACE('',(#2684),#1516,.T.);
#16413=ADVANCED_FACE('',(#2685),#933,.T.);
#16414=ADVANCED_FACE('',(#2686),#934,.T.);
#16415=ADVANCED_FACE('',(#2687),#1785,.T.);
#16416=ADVANCED_FACE('',(#2688,#1046,#1047),#1517,.F.);
#16417=ADVANCED_FACE('',(#2689),#1518,.T.);
#16418=ADVANCED_FACE('',(#2690),#935,.T.);
#16419=ADVANCED_FACE('',(#2691),#936,.T.);
#16420=ADVANCED_FACE('',(#2692),#937,.T.);
#16421=ADVANCED_FACE('',(#2693),#1519,.T.);
#16422=ADVANCED_FACE('',(#2694),#938,.T.);
#16423=ADVANCED_FACE('',(#2695),#1786,.T.);
#16424=ADVANCED_FACE('',(#2696),#1787,.T.);
#16425=ADVANCED_FACE('',(#2697),#1788,.T.);
#16426=ADVANCED_FACE('',(#2698),#1789,.T.);
#16427=ADVANCED_FACE('',(#2699),#225,.T.);
#16428=ADVANCED_FACE('',(#2700,#1048,#1049),#1520,.T.);
#16429=ADVANCED_FACE('',(#2701),#1790,.T.);
#16430=ADVANCED_FACE('',(#2702),#226,.T.);
#16431=ADVANCED_FACE('',(#2703),#1791,.T.);
#16432=ADVANCED_FACE('',(#2704),#1521,.T.);
#16433=ADVANCED_FACE('',(#2705),#1792,.T.);
#16434=ADVANCED_FACE('',(#2706),#1793,.F.);
#16435=ADVANCED_FACE('',(#2707),#1794,.F.);
#16436=ADVANCED_FACE('',(#2708),#1795,.F.);
#16437=ADVANCED_FACE('',(#2709),#1796,.F.);
#16438=ADVANCED_FACE('',(#2710),#1797,.T.);
#16439=ADVANCED_FACE('',(#2711),#227,.T.);
#16440=ADVANCED_FACE('',(#2712),#1522,.T.);
#16441=ADVANCED_FACE('',(#2713),#1523,.F.);
#16442=ADVANCED_FACE('',(#2714),#1524,.T.);
#16443=ADVANCED_FACE('',(#2715),#1525,.T.);
#16531=CLOSED_SHELL('',(#16388,#16389,#16390,#16391,#16392,#16393,#16394,
#16395,#16396,#16397,#16398,#16399,#16400,#16401,#16402,#16403,#16404,#16405,
#16406,#16407,#16408,#16409,#16410,#16411,#16412,#16413,#16414,#16415,#16416,
#16417,#16418,#16419,#16420,#16421,#16422,#16423,#16424,#16425,#16426,#16427,
#16428,#16429,#16430,#16431,#16432,#16433,#16434,#16435,#16436,#16437,#16438,
#16439,#16440,#16441,#16442,#16443));
#17879=AXIS2_PLACEMENT_3D('',#43863,#21511,#21512);
#17880=AXIS2_PLACEMENT_3D('',#43864,#21513,#21514);
#17881=AXIS2_PLACEMENT_3D('',#43873,#21519,#21520);
#17882=AXIS2_PLACEMENT_3D('',#43879,#21524,#21525);
#17883=AXIS2_PLACEMENT_3D('',#43888,#21530,#21531);
#17884=AXIS2_PLACEMENT_3D('',#43894,#21535,#21536);
#17885=AXIS2_PLACEMENT_3D('',#43905,#21542,#21543);
#17886=AXIS2_PLACEMENT_3D('',#43911,#21547,#21548);
#17887=AXIS2_PLACEMENT_3D('',#43914,#21550,#21551);
#17888=AXIS2_PLACEMENT_3D('',#43915,#21552,#21553);
#17889=AXIS2_PLACEMENT_3D('',#43916,#21554,#21555);
#17890=AXIS2_PLACEMENT_3D('',#43920,#21558,#21559);
#17891=AXIS2_PLACEMENT_3D('',#43924,#21562,#21563);
#17892=AXIS2_PLACEMENT_3D('',#43926,#21564,#21565);
#17893=AXIS2_PLACEMENT_3D('',#43927,#21566,#21567);
#17894=AXIS2_PLACEMENT_3D('',#43938,#21573,#21574);
#17895=AXIS2_PLACEMENT_3D('',#43944,#21578,#21579);
#17896=AXIS2_PLACEMENT_3D('',#43946,#21580,#21581);
#17897=AXIS2_PLACEMENT_3D('',#43949,#21583,#21584);
#17898=AXIS2_PLACEMENT_3D('',#43950,#21585,#21586);
#17899=AXIS2_PLACEMENT_3D('',#43953,#21589,#21590);
#17900=AXIS2_PLACEMENT_3D('',#43962,#21595,#21596);
#17901=AXIS2_PLACEMENT_3D('',#43963,#21597,#21598);
#17902=AXIS2_PLACEMENT_3D('',#43967,#21601,#21602);
#17903=AXIS2_PLACEMENT_3D('',#43971,#21605,#21606);
#17904=AXIS2_PLACEMENT_3D('',#43974,#21608,#21609);
#17905=AXIS2_PLACEMENT_3D('',#43975,#21610,#21611);
#17906=AXIS2_PLACEMENT_3D('',#43984,#21617,#21618);
#17907=AXIS2_PLACEMENT_3D('',#44175,#21621,#21622);
#17908=AXIS2_PLACEMENT_3D('',#44179,#21624,#21625);
#17909=AXIS2_PLACEMENT_3D('',#44182,#21628,#21629);
#17910=AXIS2_PLACEMENT_3D('',#44190,#21633,#21634);
#17911=AXIS2_PLACEMENT_3D('',#44195,#21637,#21638);
#17912=AXIS2_PLACEMENT_3D('',#44197,#21639,#21640);
#17913=AXIS2_PLACEMENT_3D('',#44198,#21641,#21642);
#17914=AXIS2_PLACEMENT_3D('',#44264,#21644,#21645);
#17915=AXIS2_PLACEMENT_3D('',#44266,#21646,#21647);
#17916=AXIS2_PLACEMENT_3D('',#44267,#21648,#21649);
#17917=AXIS2_PLACEMENT_3D('',#44458,#21653,#21654);
#17918=AXIS2_PLACEMENT_3D('',#44460,#21655,#21656);
#17919=AXIS2_PLACEMENT_3D('',#44462,#21658,#21659);
#17920=AXIS2_PLACEMENT_3D('',#44466,#21662,#21663);
#17921=AXIS2_PLACEMENT_3D('',#44468,#21664,#21665);
#17922=AXIS2_PLACEMENT_3D('',#44469,#21666,#21667);
#17923=AXIS2_PLACEMENT_3D('',#44761,#21673,#21674);
#17924=AXIS2_PLACEMENT_3D('',#44798,#21676,#21677);
#17925=AXIS2_PLACEMENT_3D('',#44799,#21678,#21679);
#17926=AXIS2_PLACEMENT_3D('',#44800,#21680,#21681);
#17927=AXIS2_PLACEMENT_3D('',#44803,#21683,#21684);
#17928=AXIS2_PLACEMENT_3D('',#44804,#21685,#21686);
#17929=AXIS2_PLACEMENT_3D('',#44806,#21688,#21689);
#17930=AXIS2_PLACEMENT_3D('',#44808,#21690,#21691);
#17931=AXIS2_PLACEMENT_3D('',#44810,#21693,#21694);
#17932=AXIS2_PLACEMENT_3D('',#44811,#21695,#21696);
#17933=AXIS2_PLACEMENT_3D('',#44812,#21697,#21698);
#17934=AXIS2_PLACEMENT_3D('',#44814,#21699,#21700);
#17935=AXIS2_PLACEMENT_3D('',#44816,#21701,#21702);
#17936=AXIS2_PLACEMENT_3D('',#44817,#21703,#21704);
#17937=AXIS2_PLACEMENT_3D('',#44819,#21705,#21706);
#17938=AXIS2_PLACEMENT_3D('',#44821,#21708,#21709);
#17939=AXIS2_PLACEMENT_3D('',#44823,#21710,#21711);
#17940=AXIS2_PLACEMENT_3D('',#44824,#21712,#21713);
#17941=AXIS2_PLACEMENT_3D('',#44825,#21714,#21715);
#17942=AXIS2_PLACEMENT_3D('',#44827,#21717,#21718);
#17943=AXIS2_PLACEMENT_3D('',#44830,#21721,#21722);
#17944=AXIS2_PLACEMENT_3D('',#44831,#21723,#21724);
#17945=AXIS2_PLACEMENT_3D('',#44833,#21726,#21727);
#17946=AXIS2_PLACEMENT_3D('',#44835,#21729,#21730);
#17947=AXIS2_PLACEMENT_3D('',#44837,#21732,#21733);
#17948=AXIS2_PLACEMENT_3D('',#44839,#21735,#21736);
#17949=AXIS2_PLACEMENT_3D('',#44841,#21737,#21738);
#17950=AXIS2_PLACEMENT_3D('',#44843,#21740,#21741);
#17951=AXIS2_PLACEMENT_3D('',#44844,#21742,#21743);
#17952=AXIS2_PLACEMENT_3D('',#44846,#21744,#21745);
#17953=AXIS2_PLACEMENT_3D('',#44847,#21746,#21747);
#17954=AXIS2_PLACEMENT_3D('',#44848,#21748,#21749);
#17955=AXIS2_PLACEMENT_3D('',#44849,#21750,#21751);
#17956=AXIS2_PLACEMENT_3D('',#44850,#21752,#21753);
#17957=AXIS2_PLACEMENT_3D('',#44851,#21754,#21755);
#21511=DIRECTION('axis',(0.,0.,1.));
#21512=DIRECTION('refdir',(1.,0.,0.));
#21513=DIRECTION('center_axis',(-0.707106781186549,0.,-0.707106781186546));
#21514=DIRECTION('ref_axis',(-0.707106781186546,0.,0.707106781186549));
#21515=DIRECTION('',(0.707106781186546,0.,-0.707106781186549));
#21516=DIRECTION('',(0.,1.,0.));
#21517=DIRECTION('',(-0.707106781186546,0.,0.707106781186549));
#21518=DIRECTION('',(0.,-1.,0.));
#21519=DIRECTION('center_axis',(-1.,0.,0.));
#21520=DIRECTION('ref_axis',(0.,0.,1.));
#21521=DIRECTION('',(0.,0.,-1.));
#21522=DIRECTION('',(0.,-1.,0.));
#21523=DIRECTION('',(0.,0.,1.));
#21524=DIRECTION('center_axis',(-0.707106781186549,0.,-0.707106781186546));
#21525=DIRECTION('ref_axis',(-0.707106781186546,0.,0.707106781186549));
#21526=DIRECTION('',(0.707106781186546,0.,-0.707106781186549));
#21527=DIRECTION('',(0.,1.,0.));
#21528=DIRECTION('',(-0.707106781186546,0.,0.707106781186549));
#21529=DIRECTION('',(0.,-1.,0.));
#21530=DIRECTION('center_axis',(-1.,0.,0.));
#21531=DIRECTION('ref_axis',(0.,0.,1.));
#21532=DIRECTION('',(0.,0.,-1.));
#21533=DIRECTION('',(0.,1.,0.));
#21534=DIRECTION('',(0.,0.,1.));
#21535=DIRECTION('center_axis',(0.0563883874434601,0.707106781186547,-0.704854843043252));
#21536=DIRECTION('ref_axis',(-0.996815278536125,0.,-0.07974522228289));
#21537=DIRECTION('',(0.996815278536125,0.,0.07974522228289));
#21538=DIRECTION('',(-0.996835435102578,0.0794928633517165,0.));
#21539=DIRECTION('',(-0.561362850588527,-0.561362850588533,-0.608065374740446));
#21540=DIRECTION('',(-0.996815278536125,0.,-0.07974522228289));
#21541=DIRECTION('',(-0.0282279077199712,0.706825008480088,0.706825008480088));
#21542=DIRECTION('center_axis',(0.,0.707106781186548,-0.707106781186548));
#21543=DIRECTION('ref_axis',(-1.,0.,0.));
#21544=DIRECTION('',(-1.,0.,0.));
#21545=DIRECTION('',(0.,0.707106781186547,0.707106781186547));
#21546=DIRECTION('',(1.,0.,0.));
#21547=DIRECTION('center_axis',(0.,-1.,0.));
#21548=DIRECTION('ref_axis',(0.,0.,-1.));
#21549=DIRECTION('',(0.,0.707106781186547,-0.707106781186548));
#21550=DIRECTION('center_axis',(0.,-1.,0.));
#21551=DIRECTION('ref_axis',(0.,0.,-1.));
#21552=DIRECTION('center_axis',(0.,1.,0.));
#21553=DIRECTION('ref_axis',(0.,0.,-1.));
#21554=DIRECTION('center_axis',(0.,0.707106781186548,0.707106781186548));
#21555=DIRECTION('ref_axis',(1.,0.,0.));
#21556=DIRECTION('',(0.577350269189625,-0.577350269189626,0.577350269189626));
#21557=DIRECTION('',(1.,0.,0.));
#21558=DIRECTION('center_axis',(0.,1.,0.));
#21559=DIRECTION('ref_axis',(1.,0.,0.));
#21560=DIRECTION('',(1.,0.,0.));
#21561=DIRECTION('',(1.,0.,0.));
#21562=DIRECTION('center_axis',(0.,-1.,0.));
#21563=DIRECTION('ref_axis',(1.,0.,0.));
#21564=DIRECTION('center_axis',(0.,-1.,0.));
#21565=DIRECTION('ref_axis',(1.,0.,0.));
#21566=DIRECTION('center_axis',(0.0563883874434601,-0.707106781186547,-0.704854843043252));
#21567=DIRECTION('ref_axis',(-0.996815278536125,0.,-0.07974522228289));
#21568=DIRECTION('',(0.996815278536125,0.,0.07974522228289));
#21569=DIRECTION('',(0.561362850588529,-0.561362850588532,0.608065374740446));
#21570=DIRECTION('',(0.996835435102578,0.0794928633517165,0.));
#21571=DIRECTION('',(-0.996815278536125,0.,-0.07974522228289));
#21572=DIRECTION('',(0.0282279077199586,0.706825008480088,-0.706825008480088));
#21573=DIRECTION('center_axis',(0.,-0.707106781186548,0.707106781186548));
#21574=DIRECTION('ref_axis',(1.,0.,0.));
#21575=DIRECTION('',(-0.577350269189625,-0.577350269189626,-0.577350269189626));
#21576=DIRECTION('',(-1.,0.,0.));
#21577=DIRECTION('',(0.,-0.707106781186547,-0.707106781186547));
#21578=DIRECTION('center_axis',(0.,1.,0.));
#21579=DIRECTION('ref_axis',(0.,0.,-1.));
#21580=DIRECTION('center_axis',(0.,-1.,0.));
#21581=DIRECTION('ref_axis',(0.,0.,-1.));
#21582=DIRECTION('',(0.,-0.707106781186547,0.707106781186547));
#21583=DIRECTION('center_axis',(0.,1.,0.));
#21584=DIRECTION('ref_axis',(0.,0.,-1.));
#21585=DIRECTION('center_axis',(0.,-0.707106781186548,-0.707106781186548));
#21586=DIRECTION('ref_axis',(-1.,0.,0.));
#21587=DIRECTION('',(-1.,0.,0.));
#21588=DIRECTION('',(1.,0.,0.));
#21589=DIRECTION('center_axis',(0.734760240582904,0.,-0.678326904124075));
#21590=DIRECTION('ref_axis',(-0.678326904124075,0.,-0.734760240582904));
#21591=DIRECTION('',(0.,1.,0.));
#21592=DIRECTION('',(0.,1.,0.));
#21593=DIRECTION('',(-0.678326904124075,0.,-0.734760240582904));
#21594=DIRECTION('',(0.,-1.,0.));
#21595=DIRECTION('center_axis',(0.734760240582904,0.,-0.678326904124075));
#21596=DIRECTION('ref_axis',(-0.678326904124075,0.,-0.734760240582904));
#21597=DIRECTION('center_axis',(0.07974522228289,0.,-0.996815278536125));
#21598=DIRECTION('ref_axis',(-0.996815278536125,0.,-0.07974522228289));
#21599=DIRECTION('',(0.,1.,0.));
#21600=DIRECTION('',(-0.996815278536125,0.,-0.07974522228289));
#21601=DIRECTION('center_axis',(0.,0.,-1.));
#21602=DIRECTION('ref_axis',(-1.,0.,0.));
#21603=DIRECTION('',(0.,1.,0.));
#21604=DIRECTION('',(-1.,0.,0.));
#21605=DIRECTION('center_axis',(0.,1.,0.));
#21606=DIRECTION('ref_axis',(0.,0.,-1.));
#21607=DIRECTION('',(0.,1.,0.));
#21608=DIRECTION('center_axis',(0.,1.,0.));
#21609=DIRECTION('ref_axis',(-1.,0.,-6.12323399573677E-17));
#21610=DIRECTION('center_axis',(0.,0.,1.));
#21611=DIRECTION('ref_axis',(1.,0.,0.));
#21612=DIRECTION('',(0.,-1.,0.));
#21613=DIRECTION('',(-1.,0.,0.));
#21614=DIRECTION('',(0.,-1.,0.));
#21615=DIRECTION('',(1.,0.,0.));
#21616=DIRECTION('',(0.,1.,0.));
#21617=DIRECTION('center_axis',(-0.707106781186548,0.,0.707106781186547));
#21618=DIRECTION('ref_axis',(0.707106781186547,0.,0.707106781186548));
#21619=DIRECTION('',(-0.678326904124083,0.,-0.734760240582897));
#21620=DIRECTION('',(0.678326904124076,0.,0.734760240582904));
#21621=DIRECTION('center_axis',(0.734760240582906,0.,-0.678326904124074));
#21622=DIRECTION('ref_axis',(-0.678326904124074,0.,-0.734760240582906));
#21623=DIRECTION('',(0.,1.,0.));
#21624=DIRECTION('center_axis',(0.734760240582906,0.,-0.678326904124074));
#21625=DIRECTION('ref_axis',(-0.678326904124074,0.,-0.734760240582906));
#21626=DIRECTION('',(0.,-1.,0.));
#21627=DIRECTION('',(0.,1.,0.));
#21628=DIRECTION('center_axis',(0.,1.,0.));
#21629=DIRECTION('ref_axis',(1.,0.,0.));
#21630=DIRECTION('',(0.,0.,-1.));
#21631=DIRECTION('',(0.707106781186547,0.,-0.707106781186548));
#21632=DIRECTION('',(1.,0.,0.));
#21633=DIRECTION('center_axis',(0.,1.,0.));
#21634=DIRECTION('ref_axis',(-1.,0.,-6.12323399573677E-17));
#21635=DIRECTION('',(-1.,0.,0.));
#21636=DIRECTION('',(-0.996815278536125,0.,-0.07974522228289));
#21637=DIRECTION('center_axis',(0.,1.,0.));
#21638=DIRECTION('ref_axis',(1.,0.,0.));
#21639=DIRECTION('center_axis',(0.,1.,0.));
#21640=DIRECTION('ref_axis',(1.,0.,0.));
#21641=DIRECTION('center_axis',(0.,0.,1.));
#21642=DIRECTION('ref_axis',(0.707106781186546,-0.707106781186549,0.));
#21643=DIRECTION('',(0.,0.,1.));
#21644=DIRECTION('center_axis',(1.,0.,0.));
#21645=DIRECTION('ref_axis',(0.,0.,-1.));
#21646=DIRECTION('center_axis',(-1.,0.,0.));
#21647=DIRECTION('ref_axis',(0.,0.,-1.));
#21648=DIRECTION('center_axis',(-1.,0.,0.));
#21649=DIRECTION('ref_axis',(0.,0.,-1.));
#21650=DIRECTION('',(0.,0.,-1.));
#21651=DIRECTION('',(0.,1.,0.));
#21652=DIRECTION('',(0.678326904124078,0.,0.734760240582902));
#21653=DIRECTION('center_axis',(-0.996815278536125,0.,-0.07974522228289));
#21654=DIRECTION('ref_axis',(0.0563883874434599,0.707106781186548,-0.704854843043251));
#21655=DIRECTION('center_axis',(-0.999203502429842,0.,-0.0399043948950148));
#21656=DIRECTION('ref_axis',(0.0399043948950148,0.,-0.999203502429842));
#21657=DIRECTION('',(0.996815278536125,0.,0.07974522228289));
#21658=DIRECTION('center_axis',(0.,1.,0.));
#21659=DIRECTION('ref_axis',(1.,0.,0.));
#21660=DIRECTION('',(-1.,0.,0.));
#21661=DIRECTION('',(-1.,0.,0.));
#21662=DIRECTION('center_axis',(0.,1.,0.));
#21663=DIRECTION('ref_axis',(1.,0.,0.));
#21664=DIRECTION('center_axis',(0.,1.,0.));
#21665=DIRECTION('ref_axis',(1.,0.,0.));
#21666=DIRECTION('center_axis',(0.,0.,-1.));
#21667=DIRECTION('ref_axis',(-1.,0.,0.));
#21668=DIRECTION('',(-1.,0.,0.));
#21669=DIRECTION('',(0.,-1.,0.));
#21670=DIRECTION('',(1.,0.,0.));
#21671=DIRECTION('',(-0.707106781186542,0.,0.707106781186553));
#21672=DIRECTION('',(0.707106781186555,0.,-0.70710678118654));
#21673=DIRECTION('center_axis',(0.70710678118655,0.,0.707106781186545));
#21674=DIRECTION('ref_axis',(0.707106781186545,0.,-0.70710678118655));
#21675=DIRECTION('',(0.707106781186539,0.,-0.707106781186556));
#21676=DIRECTION('center_axis',(-1.,0.,0.));
#21677=DIRECTION('ref_axis',(0.,-0.707106781186548,0.707106781186548));
#21678=DIRECTION('center_axis',(1.,0.,0.));
#21679=DIRECTION('ref_axis',(0.,0.,1.));
#21680=DIRECTION('center_axis',(1.,0.,0.));
#21681=DIRECTION('ref_axis',(0.,0.707106781186548,0.707106781186548));
#21682=DIRECTION('',(-1.,0.,0.));
#21683=DIRECTION('center_axis',(-1.,0.,-7.96639400082368E-16));
#21684=DIRECTION('ref_axis',(-7.96639400082368E-16,0.,1.));
#21685=DIRECTION('center_axis',(0.,0.,-1.));
#21686=DIRECTION('ref_axis',(0.707106781186546,0.707106781186549,0.));
#21687=DIRECTION('',(0.,0.,1.));
#21688=DIRECTION('center_axis',(-1.,0.,0.));
#21689=DIRECTION('ref_axis',(0.,0.707106781186548,-0.707106781186548));
#21690=DIRECTION('center_axis',(1.,0.,0.));
#21691=DIRECTION('ref_axis',(0.,0.,-1.));
#21692=DIRECTION('',(1.,0.,0.));
#21693=DIRECTION('center_axis',(0.,1.,0.));
#21694=DIRECTION('ref_axis',(0.,0.,1.));
#21695=DIRECTION('center_axis',(0.,-1.,0.));
#21696=DIRECTION('ref_axis',(-1.,0.,-6.12323399573677E-17));
#21697=DIRECTION('center_axis',(0.,1.,0.));
#21698=DIRECTION('ref_axis',(1.,0.,0.));
#21699=DIRECTION('center_axis',(0.,-1.,0.));
#21700=DIRECTION('ref_axis',(1.,0.,0.));
#21701=DIRECTION('center_axis',(0.,-1.,0.));
#21702=DIRECTION('ref_axis',(1.,0.,0.));
#21703=DIRECTION('center_axis',(0.996815278536125,0.,0.07974522228289));
#21704=DIRECTION('ref_axis',(0.05638838744346,-0.707106781186549,-0.70485484304325));
#21705=DIRECTION('center_axis',(0.999203502429842,0.,0.0399043948950059));
#21706=DIRECTION('ref_axis',(0.0399043948950059,0.,-0.999203502429842));
#21707=DIRECTION('',(0.996815278536125,0.,0.07974522228289));
#21708=DIRECTION('center_axis',(0.,-1.,0.));
#21709=DIRECTION('ref_axis',(0.,0.,-1.));
#21710=DIRECTION('center_axis',(-1.,0.,0.));
#21711=DIRECTION('ref_axis',(0.,0.,-1.));
#21712=DIRECTION('center_axis',(0.,-1.,0.));
#21713=DIRECTION('ref_axis',(-1.,0.,-6.12323399573677E-17));
#21714=DIRECTION('center_axis',(1.,0.,0.));
#21715=DIRECTION('ref_axis',(0.,-0.707106781186548,-0.707106781186548));
#21716=DIRECTION('',(1.,0.,0.));
#21717=DIRECTION('center_axis',(0.,0.,-1.));
#21718=DIRECTION('ref_axis',(1.,0.,0.));
#21719=DIRECTION('',(0.,-1.,0.));
#21720=DIRECTION('',(0.,-1.,0.));
#21721=DIRECTION('center_axis',(0.,-1.,0.));
#21722=DIRECTION('ref_axis',(0.,0.,-1.));
#21723=DIRECTION('center_axis',(0.,1.,0.));
#21724=DIRECTION('ref_axis',(1.,0.,0.));
#21725=DIRECTION('',(0.,1.,0.));
#21726=DIRECTION('center_axis',(0.,1.,0.));
#21727=DIRECTION('ref_axis',(1.,0.,0.));
#21728=DIRECTION('',(0.,1.,0.));
#21729=DIRECTION('center_axis',(0.,1.,0.));
#21730=DIRECTION('ref_axis',(1.,0.,0.));
#21731=DIRECTION('',(0.,1.,0.));
#21732=DIRECTION('center_axis',(0.,1.,0.));
#21733=DIRECTION('ref_axis',(1.,0.,0.));
#21734=DIRECTION('',(0.,1.,0.));
#21735=DIRECTION('center_axis',(1.,0.,0.));
#21736=DIRECTION('ref_axis',(0.,0.,-1.));
#21737=DIRECTION('center_axis',(1.,0.,0.));
#21738=DIRECTION('ref_axis',(0.,0.,-1.));
#21739=DIRECTION('',(-1.,0.,0.));
#21740=DIRECTION('center_axis',(1.,0.,0.));
#21741=DIRECTION('ref_axis',(0.,0.,-1.));
#21742=DIRECTION('center_axis',(0.,-1.,0.));
#21743=DIRECTION('ref_axis',(0.,0.,-1.));
#21744=DIRECTION('center_axis',(0.906307787036649,0.,0.422618261740702));
#21745=DIRECTION('ref_axis',(0.422618261740701,0.,-0.906307787036649));
#21746=DIRECTION('center_axis',(0.,1.,0.));
#21747=DIRECTION('ref_axis',(0.,0.,-1.));
#21748=DIRECTION('center_axis',(0.906307787036649,0.,0.422618261740702));
#21749=DIRECTION('ref_axis',(0.422618261740702,0.,-0.906307787036649));
#21750=DIRECTION('center_axis',(1.,0.,0.));
#21751=DIRECTION('ref_axis',(0.,0.,-1.));
#21752=DIRECTION('center_axis',(0.,0.,-1.));
#21753=DIRECTION('ref_axis',(-1.,0.,0.));
#21754=DIRECTION('center_axis',(0.07974522228289,0.,-0.996815278536125));
#21755=DIRECTION('ref_axis',(0.996815278536125,0.,0.07974522228289));
#43863=CARTESIAN_POINT('',(0.,0.,0.));
#43864=CARTESIAN_POINT('Origin',(0.249999999999999,-12.,6.75));
#43865=CARTESIAN_POINT('',(0.499999999999998,-8.1,6.5));
#43866=CARTESIAN_POINT('',(0.,-8.1,7.));
#43867=CARTESIAN_POINT('',(7.62499999999997,-8.1,-0.625000000000007));
#43868=CARTESIAN_POINT('',(0.,8.1,7.));
#43869=CARTESIAN_POINT('',(0.,-12.,7.));
#43870=CARTESIAN_POINT('',(0.499999999999998,8.1,6.5));
#43871=CARTESIAN_POINT('',(7.62499999999997,8.1,-0.625000000000007));
#43872=CARTESIAN_POINT('',(0.499999999999998,-12.,6.5));
#43873=CARTESIAN_POINT('Origin',(0.,-12.,6.5));
#43874=CARTESIAN_POINT('',(0.,-8.1,8.5));
#43875=CARTESIAN_POINT('',(0.,-8.1,3.25));
#43876=CARTESIAN_POINT('',(0.,8.1,8.5));
#43877=CARTESIAN_POINT('',(0.,-1.95,8.5));
#43878=CARTESIAN_POINT('',(0.,8.1,3.25));
#43879=CARTESIAN_POINT('Origin',(45.25,-12.,-6.75));
#43880=CARTESIAN_POINT('',(45.5,-8.1,-7.));
#43881=CARTESIAN_POINT('',(45.,-8.1,-6.5));
#43882=CARTESIAN_POINT('',(38.,-8.1,0.500000000000009));
#43883=CARTESIAN_POINT('',(45.,8.1,-6.5));
#43884=CARTESIAN_POINT('',(45.,-12.,-6.5));
#43885=CARTESIAN_POINT('',(45.5,8.1,-7.));
#43886=CARTESIAN_POINT('',(38.,8.1,0.500000000000009));
#43887=CARTESIAN_POINT('',(45.5,-12.,-7.));
#43888=CARTESIAN_POINT('Origin',(45.,-12.,-7.));
#43889=CARTESIAN_POINT('',(45.,-8.1,6.5));
#43890=CARTESIAN_POINT('',(45.,-8.1,-3.5));
#43891=CARTESIAN_POINT('',(45.,8.1,6.5));
#43892=CARTESIAN_POINT('',(45.,-12.,6.5));
#43893=CARTESIAN_POINT('',(45.,8.1,-3.5));
#43894=CARTESIAN_POINT('Origin',(26.8600318979269,-8.35,-9.00039872408616));
#43895=CARTESIAN_POINT('',(29.9800318980078,-8.1,-8.5));
#43896=CARTESIAN_POINT('',(48.7300318980078,-8.1,-7.));
#43897=CARTESIAN_POINT('',(26.8400955923562,-8.1,-8.75119490445213));
#43898=CARTESIAN_POINT('',(54.5384025518406,-8.56318980889132,-7.));
#43899=CARTESIAN_POINT('',(41.1437308530539,-7.49502873686523,-7.));
#43900=CARTESIAN_POINT('',(54.5015923607319,-8.6,-7.03987261114144));
#43901=CARTESIAN_POINT('',(51.2914447078965,-11.8101476528355,-10.5170881651225));
#43902=CARTESIAN_POINT('',(30.,-8.6,-9.));
#43903=CARTESIAN_POINT('',(26.8799682034976,-8.6,-9.24960254372019));
#43904=CARTESIAN_POINT('',(30.,-8.6,-9.));
#43905=CARTESIAN_POINT('Origin',(11.5,-8.35,-8.75));
#43906=CARTESIAN_POINT('',(0.,-8.6,-9.));
#43907=CARTESIAN_POINT('',(11.5,-8.6,-9.));
#43908=CARTESIAN_POINT('',(0.,-8.1,-8.5));
#43909=CARTESIAN_POINT('',(0.,-8.6,-9.));
#43910=CARTESIAN_POINT('',(11.5,-8.1,-8.5));
#43911=CARTESIAN_POINT('Origin',(0.,-8.35,0.));
#43912=CARTESIAN_POINT('',(0.,-8.6,9.));
#43913=CARTESIAN_POINT('',(0.,-8.6,9.));
#43914=CARTESIAN_POINT('Origin',(0.,-8.1,0.));
#43915=CARTESIAN_POINT('Origin',(0.,-8.6,0.));
#43916=CARTESIAN_POINT('Origin',(11.5,-8.35,8.75));
#43917=CARTESIAN_POINT('',(0.499999999999998,-8.6,9.));
#43918=CARTESIAN_POINT('',(1.05833333333333,-9.15833333333333,9.55833333333333));
#43919=CARTESIAN_POINT('',(11.5,-8.6,9.));
#43920=CARTESIAN_POINT('Origin',(23.,-8.1,0.));
#43921=CARTESIAN_POINT('',(34.,-8.1,6.5));
#43922=CARTESIAN_POINT('',(39.,-8.1,-7.));
#43923=CARTESIAN_POINT('',(12.95,-8.1,-2.));
#43924=CARTESIAN_POINT('Origin',(16.,-8.1,-2.));
#43925=CARTESIAN_POINT('',(-3.05,-8.1,-3.73517273739943E-16));
#43926=CARTESIAN_POINT('Origin',(0.,-8.1,0.));
#43927=CARTESIAN_POINT('Origin',(39.3600318979269,8.35,-8.00039872408616));
#43928=CARTESIAN_POINT('',(30.,8.6,-9.));
#43929=CARTESIAN_POINT('',(54.5015923607319,8.6,-7.03987261114144));
#43930=CARTESIAN_POINT('',(39.3799682034976,8.6,-8.24960254372019));
#43931=CARTESIAN_POINT('',(54.5384025518406,8.56318980889132,-7.));
#43932=CARTESIAN_POINT('',(52.1553995139966,10.9461928467353,-9.58125672850473));
#43933=CARTESIAN_POINT('',(48.7300318980078,8.1,-7.));
#43934=CARTESIAN_POINT('',(46.4033407459587,7.91445749689621,-7.));
#43935=CARTESIAN_POINT('',(29.9800318980078,8.1,-8.5));
#43936=CARTESIAN_POINT('',(39.3400955923562,8.1,-7.75119490445213));
#43937=CARTESIAN_POINT('',(29.9800318980078,8.1,-8.5));
#43938=CARTESIAN_POINT('Origin',(11.5,8.35,8.75));
#43939=CARTESIAN_POINT('',(0.499999999999998,8.6,9.));
#43940=CARTESIAN_POINT('',(0.408333333333332,8.50833333333333,8.90833333333333));
#43941=CARTESIAN_POINT('',(0.,8.6,9.));
#43942=CARTESIAN_POINT('',(11.5,8.6,9.));
#43943=CARTESIAN_POINT('',(0.,8.6,9.));
#43944=CARTESIAN_POINT('Origin',(0.,8.35,0.));
#43945=CARTESIAN_POINT('',(0.,8.6,-9.));
#43946=CARTESIAN_POINT('Origin',(0.,8.6,0.));
#43947=CARTESIAN_POINT('',(0.,8.1,-8.5));
#43948=CARTESIAN_POINT('',(0.,8.6,-9.));
#43949=CARTESIAN_POINT('Origin',(0.,8.1,0.));
#43950=CARTESIAN_POINT('Origin',(26.5,8.35,-8.75));
#43951=CARTESIAN_POINT('',(26.5,8.1,-8.5));
#43952=CARTESIAN_POINT('',(26.5,8.6,-9.));
#43953=CARTESIAN_POINT('Origin',(54.750796180366,8.1,-6.76993630557072));
#43954=CARTESIAN_POINT('',(54.5384025518406,3.87298334620742,-7.));
#43955=CARTESIAN_POINT('',(54.5384025518406,-1.95,-7.));
#43956=CARTESIAN_POINT('',(54.5015923607319,11.,-7.03987261114144));
#43957=CARTESIAN_POINT('',(54.5015923607319,8.1,-7.03987261114144));
#43958=CARTESIAN_POINT('',(55.,11.,-6.5));
#43959=CARTESIAN_POINT('',(55.,11.,-6.5));
#43960=CARTESIAN_POINT('',(55.,4.66368952654441,-6.5));
#43961=CARTESIAN_POINT('',(55.,8.1,-6.5));
#43962=CARTESIAN_POINT('Origin',(61.0007668260719,0.,0.));
#43963=CARTESIAN_POINT('Origin',(55.,8.1,-7.));
#43964=CARTESIAN_POINT('',(30.,11.,-9.));
#43965=CARTESIAN_POINT('',(30.,8.1,-9.));
#43966=CARTESIAN_POINT('',(39.3799682034976,11.,-8.24960254372019));
#43967=CARTESIAN_POINT('Origin',(30.,8.1,-9.));
#43968=CARTESIAN_POINT('',(0.,11.,-9.));
#43969=CARTESIAN_POINT('',(0.,8.1,-9.));
#43970=CARTESIAN_POINT('',(26.5,11.,-9.));
#43971=CARTESIAN_POINT('Origin',(0.,8.1,0.));
#43972=CARTESIAN_POINT('',(0.,11.,9.));
#43973=CARTESIAN_POINT('',(0.,8.1,9.));
#43974=CARTESIAN_POINT('Origin',(0.,11.,0.));
#43975=CARTESIAN_POINT('Origin',(0.,8.1,9.));
#43976=CARTESIAN_POINT('',(0.,-11.,9.));
#43977=CARTESIAN_POINT('',(0.,-8.1,9.));
#43978=CARTESIAN_POINT('',(54.5,-11.,9.));
#43979=CARTESIAN_POINT('',(11.5,-11.,9.));
#43980=CARTESIAN_POINT('',(54.5,11.,9.));
#43981=CARTESIAN_POINT('',(54.5,8.1,9.));
#43982=CARTESIAN_POINT('',(11.5,11.,9.));
#43983=CARTESIAN_POINT('',(0.5,3.075,9.));
#43984=CARTESIAN_POINT('Origin',(0.25,-1.95,8.75));
#43985=CARTESIAN_POINT('Ctrl Pts',(53.3994258036423,-11.9970763379733,-6.20150705299425));
#43986=CARTESIAN_POINT('Ctrl Pts',(53.3983950128377,-11.9971576476841,-6.20052513988951));
#43987=CARTESIAN_POINT('Ctrl Pts',(53.3943370172609,-11.9975342948482,-6.19665654944087));
#43988=CARTESIAN_POINT('Ctrl Pts',(53.3727107131384,-11.9989014878572,-6.1758928909015));
#43989=CARTESIAN_POINT('Ctrl Pts',(53.3526536192614,-11.99969335768,-6.15650865342772));
#43990=CARTESIAN_POINT('Ctrl Pts',(53.3311081853195,-12.0000565840971,-6.13563358306537));
#43991=CARTESIAN_POINT('Ctrl Pts',(53.3270617506464,-12.,-6.1317145494215));
#43992=CARTESIAN_POINT('Ctrl Pts',(53.3260375416529,-12.,-6.13072210034901));
#43993=CARTESIAN_POINT('Ctrl Pts',(53.6250878309457,-11.9970763379733,-5.95707109672624));
#43994=CARTESIAN_POINT('Ctrl Pts',(53.624046974867,-11.9971576476841,-5.95610008627501));
#43995=CARTESIAN_POINT('Ctrl Pts',(53.6199123835538,-11.9975342948482,-5.95231446393721));
#43996=CARTESIAN_POINT('Ctrl Pts',(53.5980500288147,-11.9989014878572,-5.9318064942209));
#43997=CARTESIAN_POINT('Ctrl Pts',(53.5776596596804,-11.99969335768,-5.91278325880497));
#43998=CARTESIAN_POINT('Ctrl Pts',(53.5558687126325,-12.0000565840971,-5.89217412698611));
#43999=CARTESIAN_POINT('Ctrl Pts',(53.5517314884884,-12.,-5.88835343603374));
#44000=CARTESIAN_POINT('Ctrl Pts',(53.5506916944353,-12.,-5.88737786861835));
#44001=CARTESIAN_POINT('Ctrl Pts',(53.8507498582491,-11.9970763379733,-5.71263514045823));
#44002=CARTESIAN_POINT('Ctrl Pts',(53.8496989368963,-11.9971576476841,-5.71167503266051));
#44003=CARTESIAN_POINT('Ctrl Pts',(53.8455849036831,-11.9980545985291,-5.7078554941638));
#44004=CARTESIAN_POINT('Ctrl Pts',(53.8231265400383,-11.9984560506594,-5.68769817753873));
#44005=CARTESIAN_POINT('Ctrl Pts',(53.8026126104705,-12.0001633022127,-5.66888975818738));
#44006=CARTESIAN_POINT('Ctrl Pts',(53.7804492566119,-11.9995402969754,-5.64881168903421));
#44007=CARTESIAN_POINT('Ctrl Pts',(53.7764012263304,-12.,-5.64499232264598));
#44008=CARTESIAN_POINT('Ctrl Pts',(53.7753458472176,-12.,-5.64403363688769));
#44009=CARTESIAN_POINT('Ctrl Pts',(54.0764118855525,-11.9970763379733,-5.46819918419022));
#44010=CARTESIAN_POINT('Ctrl Pts',(54.0753508989257,-11.9971576476841,-5.46724997904601));
#44011=CARTESIAN_POINT('Ctrl Pts',(54.0711710231008,-11.9975342948482,-5.46351340866015));
#44012=CARTESIAN_POINT('Ctrl Pts',(54.048748896601,-11.9989014878572,-5.44361178085813));
#44013=CARTESIAN_POINT('Ctrl Pts',(54.0278269351149,-11.99969335768,-5.42516436356463));
#44014=CARTESIAN_POINT('Ctrl Pts',(54.0053002006183,-12.0000565840971,-5.40535223295494));
#44015=CARTESIAN_POINT('Ctrl Pts',(54.0010709641725,-12.,-5.40163120925822));
#44016=CARTESIAN_POINT('Ctrl Pts',(54.,-12.,-5.40068940515703));
#44017=CARTESIAN_POINT('',(53.3260375416529,-12.,-6.13072210034901));
#44018=CARTESIAN_POINT('',(53.3994258036423,-11.9970763379733,-6.20150705299425));
#44019=CARTESIAN_POINT('Ctrl Pts',(53.3260375416529,-12.,-6.13072210034901));
#44020=CARTESIAN_POINT('Ctrl Pts',(53.3263653917992,-12.,-6.13103978411836));
#44021=CARTESIAN_POINT('Ctrl Pts',(53.3266965241738,-11.9999998537887,-6.13136064571203));
#44022=CARTESIAN_POINT('Ctrl Pts',(53.3271049857568,-11.9999993771298,-6.1317563979681));
#44023=CARTESIAN_POINT('Ctrl Pts',(53.3275337985376,-11.9999988767218,-6.13217186819225));
#44024=CARTESIAN_POINT('Ctrl Pts',(53.3280476274129,-11.9999980172876,-6.1326696741755));
#44025=CARTESIAN_POINT('Ctrl Pts',(53.3286904259905,-11.9999961533972,-6.13329239134349));
#44026=CARTESIAN_POINT('Ctrl Pts',(53.3293756063502,-11.9999941666144,-6.13395616626162));
#44027=CARTESIAN_POINT('Ctrl Pts',(53.3302070341195,-11.9999910328059,-6.13476158745548));
#44028=CARTESIAN_POINT('Ctrl Pts',(53.3311954446607,-11.9999854611243,-6.13571905555109));
#44029=CARTESIAN_POINT('Ctrl Pts',(53.3322884658049,-11.9999792997515,-6.13677785938784));
#44030=CARTESIAN_POINT('Ctrl Pts',(53.3335730356946,-11.9999701116392,-6.13802219121803));
#44031=CARTESIAN_POINT('Ctrl Pts',(53.3350185362129,-11.9999559246679,-6.13942237194384));
#44032=CARTESIAN_POINT('Ctrl Pts',(53.3368471635251,-11.9999379774705,-6.14119366755035));
#44033=CARTESIAN_POINT('Ctrl Pts',(53.3389323869447,-11.9999118325716,-6.14321346237318));
#44034=CARTESIAN_POINT('Ctrl Pts',(53.3411513308822,-11.9998751862731,-6.14536258368008));
#44035=CARTESIAN_POINT('Ctrl Pts',(53.3434411556436,-11.9998373693639,-6.14758035543208));
#44036=CARTESIAN_POINT('Ctrl Pts',(53.345868635647,-11.9997883276492,-6.14993125395063));
#44037=CARTESIAN_POINT('Ctrl Pts',(53.3482907512442,-11.9997294435353,-6.15227641841813));
#44038=CARTESIAN_POINT('Ctrl Pts',(53.3501500681357,-11.9996842416351,-6.15407666441501));
#44039=CARTESIAN_POINT('Ctrl Pts',(53.352005417499,-11.9996333964815,-6.1558727486431));
#44040=CARTESIAN_POINT('Ctrl Pts',(53.3538165595412,-11.9995784557113,-6.15762546358553));
#44041=CARTESIAN_POINT('Ctrl Pts',(53.3554526522043,-11.9995288250425,-6.15920877620872));
#44042=CARTESIAN_POINT('Ctrl Pts',(53.3570522619671,-11.9994759318124,-6.16075630398688));
#44043=CARTESIAN_POINT('Ctrl Pts',(53.3586155616919,-11.9994203574747,-6.16226796467035));
#44044=CARTESIAN_POINT('Ctrl Pts',(53.3601422105451,-11.9993660860529,-6.16374418513686));
#44045=CARTESIAN_POINT('Ctrl Pts',(53.3616336692583,-11.9993093376916,-6.16518565842691));
#44046=CARTESIAN_POINT('Ctrl Pts',(53.3631274578893,-11.9992489493601,-6.16662838182109));
#44047=CARTESIAN_POINT('Ctrl Pts',(53.3646060851576,-11.9991891739463,-6.16805646214439));
#44048=CARTESIAN_POINT('Ctrl Pts',(53.3660934825782,-11.9991255575139,-6.16949201650793));
#44049=CARTESIAN_POINT('Ctrl Pts',(53.367618365977,-11.9990565477853,-6.17096264966601));
#44050=CARTESIAN_POINT('Ctrl Pts',(53.3692606175906,-11.9989822264713,-6.17254647547123));
#44051=CARTESIAN_POINT('Ctrl Pts',(53.3709459816506,-11.9989015996314,-6.17417063363568));
#44052=CARTESIAN_POINT('Ctrl Pts',(53.3726668563583,-11.9988143988634,-6.17582784143697));
#44053=CARTESIAN_POINT('Ctrl Pts',(53.3746429322081,-11.9987142664533,-6.17773080874758));
#44054=CARTESIAN_POINT('Ctrl Pts',(53.3766652694672,-11.9986053804691,-6.1796768086172));
#44055=CARTESIAN_POINT('Ctrl Pts',(53.378673640783,-11.9984906809933,-6.18160807869434));
#44056=CARTESIAN_POINT('Ctrl Pts',(53.381387426409,-11.9983356948179,-6.18421768227407));
#44057=CARTESIAN_POINT('Ctrl Pts',(53.3840724615807,-11.998169946725,-6.18679724506432));
#44058=CARTESIAN_POINT('Ctrl Pts',(53.3865204335424,-11.9980095903933,-6.18914727674629));
#44059=CARTESIAN_POINT('Ctrl Pts',(53.3883564125136,-11.9978893231445,-6.19090980050777));
#44060=CARTESIAN_POINT('Ctrl Pts',(53.390056605587,-11.9977724646069,-6.19254088692898));
#44061=CARTESIAN_POINT('Ctrl Pts',(53.3915493621279,-11.9976666880185,-6.19397211154302));
#44062=CARTESIAN_POINT('Ctrl Pts',(53.3928168047706,-11.9975768771518,-6.19518730977343));
#44063=CARTESIAN_POINT('Ctrl Pts',(53.3939342984045,-11.9974951565352,-6.19625804170453));
#44064=CARTESIAN_POINT('Ctrl Pts',(53.3948846855004,-11.9974244749302,-6.19716807146619));
#44065=CARTESIAN_POINT('Ctrl Pts',(53.3957785612314,-11.9973579961538,-6.19802398956728));
#44066=CARTESIAN_POINT('Ctrl Pts',(53.3965241938291,-11.9973013412632,-6.19873734940401));
#44067=CARTESIAN_POINT('Ctrl Pts',(53.397138735667,-11.9972542202014,-6.19932477155095));
#44068=CARTESIAN_POINT('Ctrl Pts',(53.3977120757812,-11.9972102583533,-6.1998728102035));
#44069=CARTESIAN_POINT('Ctrl Pts',(53.3981711596242,-11.9971746073626,-6.20031108454769));
#44070=CARTESIAN_POINT('Ctrl Pts',(53.3985618556972,-11.9971441165173,-6.20068369529959));
#44071=CARTESIAN_POINT('Ctrl Pts',(53.3988803378796,-11.9971192614149,-6.20098743494198));
#44072=CARTESIAN_POINT('Ctrl Pts',(53.3991538396393,-11.9970977907398,-6.20124798489108));
#44073=CARTESIAN_POINT('Ctrl Pts',(53.3994258036423,-11.9970763379733,-6.20150705299425));
#44074=CARTESIAN_POINT('',(54.0764118855525,-11.9970763379733,-5.46819918419022));
#44075=CARTESIAN_POINT('Ctrl Pts',(54.0764118855525,-11.9970763379733,-5.46819918419022));
#44076=CARTESIAN_POINT('Ctrl Pts',(53.8507498582491,-11.9970763379733,-5.71263514045823));
#44077=CARTESIAN_POINT('Ctrl Pts',(53.6250878309457,-11.9970763379733,-5.95707109672624));
#44078=CARTESIAN_POINT('Ctrl Pts',(53.3994258036423,-11.9970763379733,-6.20150705299425));
#44079=CARTESIAN_POINT('',(54.,-12.,-5.40068940515703));
#44080=CARTESIAN_POINT('Ctrl Pts',(54.0764118855525,-11.9970763379733,-5.46819918419022));
#44081=CARTESIAN_POINT('Ctrl Pts',(54.0760722127604,-11.9971023691181,-5.46789529802103));
#44082=CARTESIAN_POINT('Ctrl Pts',(54.0757291197379,-11.9971285176846,-5.46758838194082));
#44083=CARTESIAN_POINT('Ctrl Pts',(54.0753056420862,-11.9971604987513,-5.46721012598462));
#44084=CARTESIAN_POINT('Ctrl Pts',(54.0748610599743,-11.9971940736286,-5.46681301923949));
#44085=CARTESIAN_POINT('Ctrl Pts',(54.0743281004805,-11.9972340652564,-5.46633747933918));
#44086=CARTESIAN_POINT('Ctrl Pts',(54.0736610164599,-11.9972833371987,-5.46574298228709));
#44087=CARTESIAN_POINT('Ctrl Pts',(54.0729499354457,-11.9973358588325,-5.46510927565687));
#44088=CARTESIAN_POINT('Ctrl Pts',(54.0720867541943,-11.9973988966663,-5.46434067032571));
#44089=CARTESIAN_POINT('Ctrl Pts',(54.0710601807953,-11.9974720300366,-5.46342731950875));
#44090=CARTESIAN_POINT('Ctrl Pts',(54.0699248858634,-11.9975529087587,-5.46241723824755));
#44091=CARTESIAN_POINT('Ctrl Pts',(54.0685901907654,-11.997646056145,-5.46123051783103));
#44092=CARTESIAN_POINT('Ctrl Pts',(54.0670877245001,-11.9977470807882,-5.45989552018864));
#44093=CARTESIAN_POINT('Ctrl Pts',(54.0651863733471,-11.9978749261358,-5.45820609835923));
#44094=CARTESIAN_POINT('Ctrl Pts',(54.0630173124452,-11.9980151152307,-5.4562800918209));
#44095=CARTESIAN_POINT('Ctrl Pts',(54.0607081627339,-11.9981555585065,-5.45423127183505));
#44096=CARTESIAN_POINT('Ctrl Pts',(54.0583277577051,-11.9983003355552,-5.45211922973853));
#44097=CARTESIAN_POINT('Ctrl Pts',(54.0558034072171,-11.9984449647778,-5.44988105183916));
#44098=CARTESIAN_POINT('Ctrl Pts',(54.0532835128464,-11.9985794246122,-5.44764872916434));
#44099=CARTESIAN_POINT('Ctrl Pts',(54.0513482481033,-11.9986826890108,-5.44593431787072));
#44100=CARTESIAN_POINT('Ctrl Pts',(54.0494164611994,-11.9987800458046,-5.44422410507438));
#44101=CARTESIAN_POINT('Ctrl Pts',(54.0475300683954,-11.9988698076318,-5.44255532992866));
#44102=CARTESIAN_POINT('Ctrl Pts',(54.0458259206903,-11.9989508975359,-5.4410477757603));
#44103=CARTESIAN_POINT('Ctrl Pts',(54.0441592479608,-11.9990258356104,-5.4395744161984));
#44104=CARTESIAN_POINT('Ctrl Pts',(54.0425299575421,-11.999095192017,-5.43813518392925));
#44105=CARTESIAN_POINT('Ctrl Pts',(54.0409373737401,-11.9991629858789,-5.43672837641793));
#44106=CARTESIAN_POINT('Ctrl Pts',(54.039381101088,-11.9992254815385,-5.43535470102763));
#44107=CARTESIAN_POINT('Ctrl Pts',(54.0378220639733,-11.9992844897609,-5.43397951691513));
#44108=CARTESIAN_POINT('Ctrl Pts',(54.0362803384762,-11.9993428427535,-5.43261960290821));
#44109=CARTESIAN_POINT('Ctrl Pts',(54.0347291700889,-11.9993980271028,-5.43125225130619));
#44110=CARTESIAN_POINT('Ctrl Pts',(54.03313887087,-11.9994507567847,-5.42985104760384));
#44111=CARTESIAN_POINT('Ctrl Pts',(54.0314260532856,-11.9995075488181,-5.42834189365842));
#44112=CARTESIAN_POINT('Ctrl Pts',(54.0296682220344,-11.9995614139067,-5.42679380614295));
#44113=CARTESIAN_POINT('Ctrl Pts',(54.0278734893913,-11.9996114588124,-5.42521367241687));
#44114=CARTESIAN_POINT('Ctrl Pts',(54.0258122123109,-11.9996689361296,-5.42339886537801));
#44115=CARTESIAN_POINT('Ctrl Pts',(54.0237028433572,-11.9997212431699,-5.42154230191065));
#44116=CARTESIAN_POINT('Ctrl Pts',(54.0216083794328,-11.9997665117108,-5.41969914921859));
#44117=CARTESIAN_POINT('Ctrl Pts',(54.0187800293293,-11.9998276420462,-5.41721016812596));
#44118=CARTESIAN_POINT('Ctrl Pts',(54.0159822587379,-11.9998755281407,-5.41474862664469));
#44119=CARTESIAN_POINT('Ctrl Pts',(54.0134321223697,-11.9999097849749,-5.41250509703313));
#44120=CARTESIAN_POINT('Ctrl Pts',(54.0115195200935,-11.9999354776006,-5.41082244982447));
#44121=CARTESIAN_POINT('Ctrl Pts',(54.0097487440424,-11.9999536880558,-5.40926466739841));
#44122=CARTESIAN_POINT('Ctrl Pts',(54.0081943616607,-11.9999664256549,-5.40789727780843));
#44123=CARTESIAN_POINT('Ctrl Pts',(54.0068744527208,-11.9999772418292,-5.406736154416));
#44124=CARTESIAN_POINT('Ctrl Pts',(54.0057109990572,-11.9999841813838,-5.40571268935998));
#44125=CARTESIAN_POINT('Ctrl Pts',(54.0047218043466,-11.9999888522197,-5.40484253492563));
#44126=CARTESIAN_POINT('Ctrl Pts',(54.0037913926568,-11.9999932454907,-5.4040240895286));
#44127=CARTESIAN_POINT('Ctrl Pts',(54.0030155797099,-11.9999956573955,-5.40334165912276));
#44128=CARTESIAN_POINT('Ctrl Pts',(54.002376417312,-11.9999971763164,-5.40277945700749));
#44129=CARTESIAN_POINT('Ctrl Pts',(54.0017800846694,-11.9999985934556,-5.40225492760136));
#44130=CARTESIAN_POINT('Ctrl Pts',(54.0013028624762,-11.999999233682,-5.40183519503762));
#44131=CARTESIAN_POINT('Ctrl Pts',(54.0008968882916,-11.9999995977956,-5.40147815247162));
#44132=CARTESIAN_POINT('Ctrl Pts',(54.0005662011516,-11.9999998943852,-5.40118732268617));
#44133=CARTESIAN_POINT('Ctrl Pts',(54.0002823024135,-12.,-5.40093766142703));
#44134=CARTESIAN_POINT('Ctrl Pts',(54.,-12.,-5.40068940515703));
#44135=CARTESIAN_POINT('',(53.6630187708265,-12.,-5.76570575275302));
#44136=CARTESIAN_POINT('Ctrl Pts',(54.0764118855525,-11.9970763379733,-5.46819918419022));
#44137=CARTESIAN_POINT('Ctrl Pts',(54.3504972331451,-11.9760715488571,-5.71340795054702));
#44138=CARTESIAN_POINT('Ctrl Pts',(54.7498941157113,-11.7487468298691,-6.13435950914876));
#44139=CARTESIAN_POINT('Ctrl Pts',(54.9796857837848,-11.2917992749461,-6.46017864830904));
#44140=CARTESIAN_POINT('Ctrl Pts',(55.,-11.0939065095575,-6.5));
#44141=CARTESIAN_POINT('Ctrl Pts',(55.,-11.,-6.5));
#44142=CARTESIAN_POINT('Ctrl Pts',(53.8507498582491,-11.9970763379733,-5.71263514045823));
#44143=CARTESIAN_POINT('Ctrl Pts',(54.122235037212,-11.9760715488571,-5.96066039620419));
#44144=CARTESIAN_POINT('Ctrl Pts',(54.5389866050285,-11.748746829869,-6.36281344831557));
#44145=CARTESIAN_POINT('Ctrl Pts',(54.8065498116121,-11.2917992749461,-6.64771864973562));
#44146=CARTESIAN_POINT('Ctrl Pts',(54.833864120244,-11.0939065095575,-6.67995753704715));
#44147=CARTESIAN_POINT('Ctrl Pts',(54.833864120244,-11.,-6.67995753704715));
#44148=CARTESIAN_POINT('Ctrl Pts',(53.6250878309457,-11.9970763379733,-5.95707109672624));
#44149=CARTESIAN_POINT('Ctrl Pts',(53.893972841279,-11.9760715488571,-6.20791284186136));
#44150=CARTESIAN_POINT('Ctrl Pts',(54.3280790943458,-11.748746829869,-6.59126738748238));
#44151=CARTESIAN_POINT('Ctrl Pts',(54.6334138394395,-11.2917992749461,-6.83525865116221));
#44152=CARTESIAN_POINT('Ctrl Pts',(54.667728240488,-11.0939065095575,-6.8599150740943));
#44153=CARTESIAN_POINT('Ctrl Pts',(54.667728240488,-11.,-6.8599150740943));
#44154=CARTESIAN_POINT('Ctrl Pts',(53.3994258036423,-11.9970763379733,-6.20150705299425));
#44155=CARTESIAN_POINT('Ctrl Pts',(53.665710645346,-11.9760715488571,-6.45516528751854));
#44156=CARTESIAN_POINT('Ctrl Pts',(54.1171715836631,-11.748746829869,-6.81972132664919));
#44157=CARTESIAN_POINT('Ctrl Pts',(54.4602778672668,-11.2917992749461,-7.0227986525888));
#44158=CARTESIAN_POINT('Ctrl Pts',(54.5015923607319,-11.0939065095575,-7.03987261114145));
#44159=CARTESIAN_POINT('Ctrl Pts',(54.5015923607319,-11.,-7.03987261114145));
#44160=CARTESIAN_POINT('',(54.5015923607319,-11.,-7.03987261114145));
#44161=CARTESIAN_POINT('Ctrl Pts',(53.3994258036423,-11.9970763379733,-6.20150705299425));
#44162=CARTESIAN_POINT('Ctrl Pts',(53.665710645346,-11.9760715488571,-6.45516528751854));
#44163=CARTESIAN_POINT('Ctrl Pts',(54.1171715836631,-11.748746829869,-6.81972132664919));
#44164=CARTESIAN_POINT('Ctrl Pts',(54.4602778672668,-11.2917992749461,-7.0227986525888));
#44165=CARTESIAN_POINT('Ctrl Pts',(54.5015923607319,-11.0939065095575,-7.03987261114145));
#44166=CARTESIAN_POINT('Ctrl Pts',(54.5015923607319,-11.,-7.03987261114145));
#44167=CARTESIAN_POINT('',(55.,-11.,-6.5));
#44168=CARTESIAN_POINT('',(54.5015923607319,-11.,-7.03987261114145));
#44169=CARTESIAN_POINT('Ctrl Pts',(55.,-11.,-6.5));
#44170=CARTESIAN_POINT('Ctrl Pts',(55.,-11.0939065095575,-6.5));
#44171=CARTESIAN_POINT('Ctrl Pts',(54.9796857837848,-11.2917992749461,-6.46017864830904));
#44172=CARTESIAN_POINT('Ctrl Pts',(54.7498941157113,-11.7487468298691,-6.13435950914876));
#44173=CARTESIAN_POINT('Ctrl Pts',(54.3504972331451,-11.9760715488571,-5.71340795054702));
#44174=CARTESIAN_POINT('Ctrl Pts',(54.0764118855525,-11.9970763379733,-5.46819918419022));
#44175=CARTESIAN_POINT('Origin',(54.750796180366,0.,-6.76993630557072));
#44176=CARTESIAN_POINT('',(54.5384025518406,-3.87298334620742,-7.));
#44177=CARTESIAN_POINT('',(54.5384025518406,-6.,-7.));
#44178=CARTESIAN_POINT('',(55.,-4.66368952654441,-6.5));
#44179=CARTESIAN_POINT('Origin',(61.0007668260719,0.,0.));
#44180=CARTESIAN_POINT('',(55.,0.,-6.5));
#44181=CARTESIAN_POINT('',(54.5015923607319,0.,-7.03987261114144));
#44182=CARTESIAN_POINT('Origin',(23.,-12.,0.));
#44183=CARTESIAN_POINT('',(54.,-12.,7.29826682694392));
#44184=CARTESIAN_POINT('',(54.,-12.,4.5));
#44185=CARTESIAN_POINT('',(53.2982668269439,-12.,8.));
#44186=CARTESIAN_POINT('',(53.649133413472,-12.,7.64913341347196));
#44187=CARTESIAN_POINT('',(0.,-12.,8.));
#44188=CARTESIAN_POINT('',(11.5,-12.,8.));
#44189=CARTESIAN_POINT('',(0.,-12.,-8.));
#44190=CARTESIAN_POINT('Origin',(0.,-12.,0.));
#44191=CARTESIAN_POINT('',(29.9600637960156,-12.,-8.));
#44192=CARTESIAN_POINT('',(11.5,-12.,-8.));
#44193=CARTESIAN_POINT('',(26.8002229812147,-12.,-8.25278726518407));
#44194=CARTESIAN_POINT('',(12.95,-12.,-2.));
#44195=CARTESIAN_POINT('Origin',(16.,-12.,-2.));
#44196=CARTESIAN_POINT('',(-3.05,-12.,3.73517273739943E-16));
#44197=CARTESIAN_POINT('Origin',(0.,-12.,0.));
#44198=CARTESIAN_POINT('Origin',(54.,-11.,4.5));
#44199=CARTESIAN_POINT('',(55.,-11.,8.5));
#44200=CARTESIAN_POINT('',(55.,-11.,4.5));
#44201=CARTESIAN_POINT('',(54.0739345923054,-11.9972630926995,7.36867780326845));
#44202=CARTESIAN_POINT('Ctrl Pts',(54.0739345923054,-11.9972630926995,7.36867780326845));
#44203=CARTESIAN_POINT('Ctrl Pts',(54.3510337690789,-11.9767196525453,7.63593113286991));
#44204=CARTESIAN_POINT('Ctrl Pts',(54.7553166986942,-11.7446620906573,8.09873418111303));
#44205=CARTESIAN_POINT('Ctrl Pts',(54.9514928044654,-11.3451725484552,8.40875696033662));
#44206=CARTESIAN_POINT('Ctrl Pts',(54.9944234105006,-11.1325383755072,8.488654852558));
#44207=CARTESIAN_POINT('Ctrl Pts',(55.,-11.0439996496616,8.5));
#44208=CARTESIAN_POINT('Ctrl Pts',(55.,-11.,8.5));
#44209=CARTESIAN_POINT('Ctrl Pts',(54.,-12.,7.29826682694392));
#44210=CARTESIAN_POINT('Ctrl Pts',(54.0003314977971,-12.,7.29858113228725));
#44211=CARTESIAN_POINT('Ctrl Pts',(54.0006663098912,-11.9999998632791,7.29889858217632));
#44212=CARTESIAN_POINT('Ctrl Pts',(54.0010792590121,-11.9999994175998,7.29929014342446));
#44213=CARTESIAN_POINT('Ctrl Pts',(54.0015127758868,-11.9999989497226,7.29970120716084));
#44214=CARTESIAN_POINT('Ctrl Pts',(54.0020321949842,-11.9999981461834,7.30019374676313));
#44215=CARTESIAN_POINT('Ctrl Pts',(54.0026819516524,-11.9999964035612,7.30080989895442));
#44216=CARTESIAN_POINT('Ctrl Pts',(54.0033745293584,-11.9999945460946,7.30146665754134));
#44217=CARTESIAN_POINT('Ctrl Pts',(54.0042148986562,-11.9999916163369,7.3022635810719));
#44218=CARTESIAN_POINT('Ctrl Pts',(54.0052139420484,-11.9999864073118,7.30321098451133));
#44219=CARTESIAN_POINT('Ctrl Pts',(54.0063186100511,-11.9999806475585,7.30425855288863));
#44220=CARTESIAN_POINT('Ctrl Pts',(54.0076168538779,-11.9999720586087,7.30548969855211));
#44221=CARTESIAN_POINT('Ctrl Pts',(54.0090777731715,-11.9999587961682,7.30687513396345));
#44222=CARTESIAN_POINT('Ctrl Pts',(54.0109250805974,-11.9999420260395,7.30862699331299));
#44223=CARTESIAN_POINT('Ctrl Pts',(54.0130315429888,-11.9999175989922,7.31062464255686));
#44224=CARTESIAN_POINT('Ctrl Pts',(54.0152731305057,-11.9998833589397,7.31275060112912));
#44225=CARTESIAN_POINT('Ctrl Pts',(54.0175900257341,-11.9998479685685,7.31494798277705));
#44226=CARTESIAN_POINT('Ctrl Pts',(54.0200464787717,-11.9998020541947,7.31727788628092));
#44227=CARTESIAN_POINT('Ctrl Pts',(54.0224971606944,-11.9997469068523,7.31960281446228));
#44228=CARTESIAN_POINT('Ctrl Pts',(54.0243769090201,-11.9997046071464,7.32138610580481));
#44229=CARTESIAN_POINT('Ctrl Pts',(54.0262524447249,-11.9996570221597,7.3231656968352));
#44230=CARTESIAN_POINT('Ctrl Pts',(54.0280827898051,-11.999605600683,7.32490295874137));
#44231=CARTESIAN_POINT('Ctrl Pts',(54.0297361262051,-11.9995591520651,7.32647221383799));
#44232=CARTESIAN_POINT('Ctrl Pts',(54.0313521786804,-11.9995096475949,7.32800653980115));
#44233=CARTESIAN_POINT('Ctrl Pts',(54.032930797643,-11.999457634203,7.32950604809328));
#44234=CARTESIAN_POINT('Ctrl Pts',(54.0344384154927,-11.9994079602032,7.33093811341151));
#44235=CARTESIAN_POINT('Ctrl Pts',(54.0359114872389,-11.9993560618632,7.33233803713807));
#44236=CARTESIAN_POINT('Ctrl Pts',(54.037384667835,-11.9993009489693,7.33373900926913));
#44237=CARTESIAN_POINT('Ctrl Pts',(54.0388731910723,-11.9992452620945,7.33515457201643));
#44238=CARTESIAN_POINT('Ctrl Pts',(54.0403683295817,-11.9991860424168,7.33657740804058));
#44239=CARTESIAN_POINT('Ctrl Pts',(54.0418997567846,-11.9991218195903,7.33803587655173));
#44240=CARTESIAN_POINT('Ctrl Pts',(54.0435473954296,-11.9990527232527,7.33960502007804));
#44241=CARTESIAN_POINT('Ctrl Pts',(54.0452366728309,-11.9989777892673,7.34121506113945));
#44242=CARTESIAN_POINT('Ctrl Pts',(54.0469610411776,-11.9988967216942,7.34285972054902));
#44243=CARTESIAN_POINT('Ctrl Pts',(54.0489358739595,-11.9988038790594,7.34474326667384));
#44244=CARTESIAN_POINT('Ctrl Pts',(54.050956174741,-11.9987029134817,7.34667169080142));
#44245=CARTESIAN_POINT('Ctrl Pts',(54.0529636122053,-11.9985964429048,7.34858912507421));
#44246=CARTESIAN_POINT('Ctrl Pts',(54.0557063045387,-11.9984509758403,7.35120884916192));
#44247=CARTESIAN_POINT('Ctrl Pts',(54.0584218496309,-11.9982950689308,7.35380508415633));
#44248=CARTESIAN_POINT('Ctrl Pts',(54.0608986078143,-11.998143957336,7.3561748403444));
#44249=CARTESIAN_POINT('Ctrl Pts',(54.0627561764518,-11.9980306236398,7.35795215748545));
#44250=CARTESIAN_POINT('Ctrl Pts',(54.0644768750634,-11.9979203495853,7.35959962417965));
#44251=CARTESIAN_POINT('Ctrl Pts',(54.0659873571994,-11.9978204591458,7.36104670175641));
#44252=CARTESIAN_POINT('Ctrl Pts',(54.0672641265468,-11.997736024482,7.36226987695943));
#44253=CARTESIAN_POINT('Ctrl Pts',(54.0683903006567,-11.9976591045265,7.36334949002639));
#44254=CARTESIAN_POINT('Ctrl Pts',(54.069348232894,-11.9975925133011,7.36426842264621));
#44255=CARTESIAN_POINT('Ctrl Pts',(54.0702488889839,-11.997529903661,7.36513241096188));
#44256=CARTESIAN_POINT('Ctrl Pts',(54.0710004010606,-11.99747648006,7.36585395496795));
#44257=CARTESIAN_POINT('Ctrl Pts',(54.0716194711387,-11.9974320284379,7.36644887928455));
#44258=CARTESIAN_POINT('Ctrl Pts',(54.0721967381906,-11.9973905784345,7.3670036310299));
#44259=CARTESIAN_POINT('Ctrl Pts',(54.0726586923053,-11.9973569415986,7.36744813846609));
#44260=CARTESIAN_POINT('Ctrl Pts',(54.0730507354953,-11.9973282258332,7.36782577118979));
#44261=CARTESIAN_POINT('Ctrl Pts',(54.0733781629767,-11.997304242938,7.36814116330667));
#44262=CARTESIAN_POINT('Ctrl Pts',(54.0736572293399,-11.9972836556963,7.36841029552303));
#44263=CARTESIAN_POINT('Ctrl Pts',(54.0739345923054,-11.9972630926995,7.36867780326845));
#44264=CARTESIAN_POINT('Origin',(55.,8.1,9.));
#44265=CARTESIAN_POINT('',(55.,-9.79717439317883E-16,8.));
#44266=CARTESIAN_POINT('Origin',(55.,0.,0.));
#44267=CARTESIAN_POINT('Origin',(55.,0.,0.));
#44268=CARTESIAN_POINT('',(55.,11.,8.5));
#44269=CARTESIAN_POINT('',(55.,11.,4.5));
#44270=CARTESIAN_POINT('',(55.,8.1,8.5));
#44271=CARTESIAN_POINT('Ctrl Pts',(54.0764118855525,11.9970763379733,-5.46819918419023));
#44272=CARTESIAN_POINT('Ctrl Pts',(54.0753508989257,11.9971576476841,-5.46724997904602));
#44273=CARTESIAN_POINT('Ctrl Pts',(54.0711710231008,11.9975342948482,-5.46351340866014));
#44274=CARTESIAN_POINT('Ctrl Pts',(54.048748896601,11.9989014878572,-5.44361178085813));
#44275=CARTESIAN_POINT('Ctrl Pts',(54.0278269351149,11.99969335768,-5.42516436356463));
#44276=CARTESIAN_POINT('Ctrl Pts',(54.0053002006183,12.0000565840971,-5.40535223295495));
#44277=CARTESIAN_POINT('Ctrl Pts',(54.0010709641725,12.,-5.40163120925821));
#44278=CARTESIAN_POINT('Ctrl Pts',(54.,12.,-5.40068940515702));
#44279=CARTESIAN_POINT('Ctrl Pts',(53.8507498582491,11.9970763379733,-5.71263514045823));
#44280=CARTESIAN_POINT('Ctrl Pts',(53.8496989368964,11.9971576476841,-5.71167503266052));
#44281=CARTESIAN_POINT('Ctrl Pts',(53.8455956568079,11.9975342948482,-5.7078554941638));
#44282=CARTESIAN_POINT('Ctrl Pts',(53.8234095809246,11.9989014878572,-5.68769817753873));
#44283=CARTESIAN_POINT('Ctrl Pts',(53.8028208946958,11.99969335768,-5.66888975818739));
#44284=CARTESIAN_POINT('Ctrl Pts',(53.7805396733053,12.0000565840971,-5.64881168903421));
#44285=CARTESIAN_POINT('Ctrl Pts',(53.7764012263304,12.,-5.64499232264597));
#44286=CARTESIAN_POINT('Ctrl Pts',(53.7753458472177,12.,-5.64403363688768));
#44287=CARTESIAN_POINT('Ctrl Pts',(53.6250878309457,11.9970763379733,-5.95707109672624));
#44288=CARTESIAN_POINT('Ctrl Pts',(53.624046974867,11.9971576476841,-5.95610008627502));
#44289=CARTESIAN_POINT('Ctrl Pts',(53.6199115260435,11.9980545985291,-5.9523037450581));
#44290=CARTESIAN_POINT('Ctrl Pts',(53.5980274576563,11.9984560506594,-5.93152435474098));
#44291=CARTESIAN_POINT('Ctrl Pts',(53.5776430500085,12.0001633022127,-5.91257563790681));
#44292=CARTESIAN_POINT('Ctrl Pts',(53.5558615023331,11.9995402969754,-5.8920839982447));
#44293=CARTESIAN_POINT('Ctrl Pts',(53.5517314884884,12.,-5.88835343603373));
#44294=CARTESIAN_POINT('Ctrl Pts',(53.5506916944353,12.,-5.88737786861835));
#44295=CARTESIAN_POINT('Ctrl Pts',(53.3994258036423,11.9970763379733,-6.20150705299425));
#44296=CARTESIAN_POINT('Ctrl Pts',(53.3983950128377,11.9971576476841,-6.20052513988952));
#44297=CARTESIAN_POINT('Ctrl Pts',(53.3943370172609,11.9975342948482,-6.19665654944088));
#44298=CARTESIAN_POINT('Ctrl Pts',(53.3727107131384,11.9989014878572,-6.17589289090149));
#44299=CARTESIAN_POINT('Ctrl Pts',(53.3526536192614,11.99969335768,-6.15650865342773));
#44300=CARTESIAN_POINT('Ctrl Pts',(53.3311081853195,12.0000565840971,-6.13563358306537));
#44301=CARTESIAN_POINT('Ctrl Pts',(53.3270617506464,12.,-6.13171454942149));
#44302=CARTESIAN_POINT('Ctrl Pts',(53.3260375416529,12.,-6.13072210034901));
#44303=CARTESIAN_POINT('',(54.,12.,-5.40068940515702));
#44304=CARTESIAN_POINT('',(54.0764118855525,11.9970763379733,-5.46819918419023));
#44305=CARTESIAN_POINT('Ctrl Pts',(54.,12.,-5.40068940515702));
#44306=CARTESIAN_POINT('Ctrl Pts',(54.0003428165178,12.,-5.40099087742915));
#44307=CARTESIAN_POINT('Ctrl Pts',(54.0006890624815,11.9999998537887,-5.40129536806019));
#44308=CARTESIAN_POINT('Ctrl Pts',(54.0011161272366,11.9999993771298,-5.40167096945517));
#44309=CARTESIAN_POINT('Ctrl Pts',(54.0015644700743,11.9999988767218,-5.40206528482136));
#44310=CARTESIAN_POINT('Ctrl Pts',(54.0021016660821,11.9999980172876,-5.40253777964602));
#44311=CARTESIAN_POINT('Ctrl Pts',(54.0027736601848,11.9999961533972,-5.4031288723702));
#44312=CARTESIAN_POINT('Ctrl Pts',(54.0034899610248,11.9999941666144,-5.40375893774298));
#44313=CARTESIAN_POINT('Ctrl Pts',(54.0043591195687,11.9999910328059,-5.40452348915422));
#44314=CARTESIAN_POINT('Ctrl Pts',(54.0053923594135,11.9999854611243,-5.40543239837707));
#44315=CARTESIAN_POINT('Ctrl Pts',(54.006534954469,11.9999792997515,-5.40643750400599));
#44316=CARTESIAN_POINT('Ctrl Pts',(54.0078777617603,11.9999701116392,-5.40761875337999));
#44317=CARTESIAN_POINT('Ctrl Pts',(54.0093887550606,11.9999559246679,-5.40894799265849));
#44318=CARTESIAN_POINT('Ctrl Pts',(54.0113002338754,11.9999379774705,-5.41062954394014));
#44319=CARTESIAN_POINT('Ctrl Pts',(54.0134798828194,11.9999118325716,-5.41254705751686));
#44320=CARTESIAN_POINT('Ctrl Pts',(54.015799109951,11.9998751862731,-5.41458755257959));
#44321=CARTESIAN_POINT('Ctrl Pts',(54.0181924213024,11.9998373693639,-5.41669322818569));
#44322=CARTESIAN_POINT('Ctrl Pts',(54.0207294127965,11.9997883276492,-5.41892550441653));
#44323=CARTESIAN_POINT('Ctrl Pts',(54.0232602607152,11.9997294435353,-5.42115289058855));
#44324=CARTESIAN_POINT('Ctrl Pts',(54.0252030450688,11.9996842416351,-5.42286272505649));
#44325=CARTESIAN_POINT('Ctrl Pts',(54.0271413645163,11.9996333964815,-5.42456893651285));
#44326=CARTESIAN_POINT('Ctrl Pts',(54.0290329274746,11.9995784557113,-5.42623453992945));
#44327=CARTESIAN_POINT('Ctrl Pts',(54.0307416682612,11.9995288250425,-5.42773916047606));
#44328=CARTESIAN_POINT('Ctrl Pts',(54.0324118288305,11.9994759318124,-5.42921026798065));
#44329=CARTESIAN_POINT('Ctrl Pts',(54.0340433409798,11.9994203574747,-5.43064804131396));
#44330=CARTESIAN_POINT('Ctrl Pts',(54.0356366030475,11.9993660860529,-5.43205210668668));
#44331=CARTESIAN_POINT('Ctrl Pts',(54.0371924223533,11.9993093376916,-5.4334238649114));
#44332=CARTESIAN_POINT('Ctrl Pts',(54.0387496735818,11.9992489493601,-5.43479784594404));
#44333=CARTESIAN_POINT('Ctrl Pts',(54.0402911193272,11.9991891739463,-5.43615788161346));
#44334=CARTESIAN_POINT('Ctrl Pts',(54.0418407146879,11.9991255575138,-5.43752606348578));
#44335=CARTESIAN_POINT('Ctrl Pts',(54.0434282664545,11.9990565477853,-5.43892881458755));
#44336=CARTESIAN_POINT('Ctrl Pts',(54.0451380099357,11.9989822264713,-5.44043953354628));
#44337=CARTESIAN_POINT('Ctrl Pts',(54.0468913953403,11.9989015996314,-5.44199001133725));
#44338=CARTESIAN_POINT('Ctrl Pts',(54.0486805569323,11.9988143988633,-5.44357325113376));
#44339=CARTESIAN_POINT('Ctrl Pts',(54.05073504643,11.9987142664533,-5.44539128118125));
#44340=CARTESIAN_POINT('Ctrl Pts',(54.0528361205663,11.9986053804691,-5.44725199366727));
#44341=CARTESIAN_POINT('Ctrl Pts',(54.0549213981032,11.9984906809933,-5.44909995931825));
#44342=CARTESIAN_POINT('Ctrl Pts',(54.0577391022603,11.9983356948179,-5.45159699887533));
#44343=CARTESIAN_POINT('Ctrl Pts',(54.0605245685882,11.998169946725,-5.45406777514985));
#44344=CARTESIAN_POINT('Ctrl Pts',(54.0630623301421,11.9980095903933,-5.45632054720379));
#44345=CARTESIAN_POINT('Ctrl Pts',(54.0649656513074,11.9978893231445,-5.45801012624424));
#44346=CARTESIAN_POINT('Ctrl Pts',(54.0667271254473,11.9977724646069,-5.45957483332706));
#44347=CARTESIAN_POINT('Ctrl Pts',(54.0682728322117,11.9976666880185,-5.4609487025292));
#44348=CARTESIAN_POINT('Ctrl Pts',(54.0695852328695,11.9975768771518,-5.46211520246701));
#44349=CARTESIAN_POINT('Ctrl Pts',(54.0707416695959,11.9974951565352,-5.46314375143915));
#44350=CARTESIAN_POINT('Ctrl Pts',(54.0717245899964,11.9974244749302,-5.46401854129122));
#44351=CARTESIAN_POINT('Ctrl Pts',(54.0726490645556,11.9973579961537,-5.46484131489773));
#44352=CARTESIAN_POINT('Ctrl Pts',(54.0734196131772,11.9973013412632,-5.46552768582455));
#44353=CARTESIAN_POINT('Ctrl Pts',(54.0740541713237,11.9972542202014,-5.46609342640823));
#44354=CARTESIAN_POINT('Ctrl Pts',(54.0746461857607,11.9972102583533,-5.46662123712968));
#44355=CARTESIAN_POINT('Ctrl Pts',(54.0751196740662,11.9971746073626,-5.46704390863355));
#44356=CARTESIAN_POINT('Ctrl Pts',(54.0755222543019,11.9971441165173,-5.46740364652107));
#44357=CARTESIAN_POINT('Ctrl Pts',(54.0758504240505,11.9971192614149,-5.46769689264119));
#44358=CARTESIAN_POINT('Ctrl Pts',(54.0761319546792,11.9970977907398,-5.46794874576034));
#44359=CARTESIAN_POINT('Ctrl Pts',(54.0764118855525,11.9970763379733,-5.46819918419023));
#44360=CARTESIAN_POINT('',(53.3994258036423,11.9970763379733,-6.20150705299425));
#44361=CARTESIAN_POINT('Ctrl Pts',(53.3994258036423,11.9970763379733,-6.20150705299425));
#44362=CARTESIAN_POINT('Ctrl Pts',(53.6250878309457,11.9970763379733,-5.95707109672624));
#44363=CARTESIAN_POINT('Ctrl Pts',(53.8507498582491,11.9970763379733,-5.71263514045823));
#44364=CARTESIAN_POINT('Ctrl Pts',(54.0764118855525,11.9970763379733,-5.46819918419023));
#44365=CARTESIAN_POINT('',(53.3260375416529,12.,-6.13072210034901));
#44366=CARTESIAN_POINT('Ctrl Pts',(53.3994258036423,11.9970763379733,-6.20150705299425));
#44367=CARTESIAN_POINT('Ctrl Pts',(53.3990957979836,11.9971023691181,-6.20119269543551));
#44368=CARTESIAN_POINT('Ctrl Pts',(53.3987624993162,11.9971285176846,-6.20087517015968));
#44369=CARTESIAN_POINT('Ctrl Pts',(53.3983516776804,11.9971604987513,-6.20048320527172));
#44370=CARTESIAN_POINT('Ctrl Pts',(53.3979203823103,11.9971940736286,-6.2000717063956));
#44371=CARTESIAN_POINT('Ctrl Pts',(53.3974038558988,11.9972340652564,-6.19957836626438));
#44372=CARTESIAN_POINT('Ctrl Pts',(53.3967580553908,11.9972833371987,-6.19896081502021));
#44373=CARTESIAN_POINT('Ctrl Pts',(53.3960696616261,11.9973358588325,-6.19830253367709));
#44374=CARTESIAN_POINT('Ctrl Pts',(53.3952346695081,11.9973988966663,-6.19750339402051));
#44375=CARTESIAN_POINT('Ctrl Pts',(53.3942423631352,11.9974720300366,-6.19655292533578));
#44376=CARTESIAN_POINT('Ctrl Pts',(53.3931449643548,11.9975529087587,-6.19550179515672));
#44377=CARTESIAN_POINT('Ctrl Pts',(53.391855587755,11.997646056145,-6.19426598597423));
#44378=CARTESIAN_POINT('Ctrl Pts',(53.390405027202,11.9977470807882,-6.19287476432927));
#44379=CARTESIAN_POINT('Ctrl Pts',(53.3885693620402,11.9978749261358,-6.19111419176947));
#44380=CARTESIAN_POINT('Ctrl Pts',(53.3864765170525,11.9980151152307,-6.18910562854187));
#44381=CARTESIAN_POINT('Ctrl Pts',(53.3842500783306,11.9981555585065,-6.18696721643439));
#44382=CARTESIAN_POINT('Ctrl Pts',(53.3819549365717,11.9983003355552,-6.18476281759905));
#44383=CARTESIAN_POINT('Ctrl Pts',(53.3795225817548,11.9984449647777,-6.18242499045831));
#44384=CARTESIAN_POINT('Ctrl Pts',(53.3770964188692,11.9985794246121,-6.18009113831728));
#44385=CARTESIAN_POINT('Ctrl Pts',(53.3752331393809,11.9986826890108,-6.17829875296305));
#44386=CARTESIAN_POINT('Ctrl Pts',(53.3733743223599,11.9987800458046,-6.17650949956189));
#44387=CARTESIAN_POINT('Ctrl Pts',(53.3715604309847,11.9988698076318,-6.17476219123845));
#44388=CARTESIAN_POINT('Ctrl Pts',(53.3699217803189,11.9989508975359,-6.1731836910114));
#44389=CARTESIAN_POINT('Ctrl Pts',(53.3683202038096,11.9990258356104,-6.17163981955613));
#44390=CARTESIAN_POINT('Ctrl Pts',(53.3667556269677,11.999095192017,-6.17013048987079));
#44391=CARTESIAN_POINT('Ctrl Pts',(53.3652262987972,11.9991629858789,-6.16865516418234));
#44392=CARTESIAN_POINT('Ctrl Pts',(53.3637328928719,11.9992254815385,-6.16721339187455));
#44393=CARTESIAN_POINT('Ctrl Pts',(53.3622377625765,11.9992844897609,-6.1657689842216));
#44394=CARTESIAN_POINT('Ctrl Pts',(53.3607592342745,11.9993428427535,-6.16434061533548));
#44395=CARTESIAN_POINT('Ctrl Pts',(53.3592725390386,11.9993980271028,-6.16290342674496));
#44396=CARTESIAN_POINT('Ctrl Pts',(53.3577489790151,11.9994507567847,-6.1614299314868));
#44397=CARTESIAN_POINT('Ctrl Pts',(53.3561080422857,11.9995075488181,-6.15984291656622));
#44398=CARTESIAN_POINT('Ctrl Pts',(53.3544247063539,11.9995614139066,-6.15821413610097));
#44399=CARTESIAN_POINT('Ctrl Pts',(53.3527064835601,11.9996114588124,-6.15655112729673));
#44400=CARTESIAN_POINT('Ctrl Pts',(53.3507330791772,11.9996689361296,-6.15464113700044));
#44401=CARTESIAN_POINT('Ctrl Pts',(53.3487142162513,11.9997212431699,-6.15268653786576));
#44402=CARTESIAN_POINT('Ctrl Pts',(53.346709909996,11.9997665117107,-6.15074572684662));
#44403=CARTESIAN_POINT('Ctrl Pts',(53.3440033082071,11.9998276420462,-6.14812486860091));
#44404=CARTESIAN_POINT('Ctrl Pts',(53.3413264972121,11.9998755281407,-6.14553230430206));
#44405=CARTESIAN_POINT('Ctrl Pts',(53.3388867514259,11.9999097849749,-6.14316920017543));
#44406=CARTESIAN_POINT('Ctrl Pts',(53.3370569420862,11.9999354776006,-6.14139687208045));
#44407=CARTESIAN_POINT('Ctrl Pts',(53.3353629098334,11.9999536880558,-6.1397559611636));
#44408=CARTESIAN_POINT('Ctrl Pts',(53.3338759204298,11.9999664256549,-6.13831557184363));
#44409=CARTESIAN_POINT('Ctrl Pts',(53.3326132384602,11.9999772418292,-6.13709246048908));
#44410=CARTESIAN_POINT('Ctrl Pts',(53.3315002529843,11.9999841813838,-6.13601432854974));
#44411=CARTESIAN_POINT('Ctrl Pts',(53.3305539861973,11.9999888522197,-6.1350976748075));
#44412=CARTESIAN_POINT('Ctrl Pts',(53.3296639514339,11.9999932454907,-6.13423549332984));
#44413=CARTESIAN_POINT('Ctrl Pts',(53.3289218270029,11.9999956573955,-6.13351657169551));
#44414=CARTESIAN_POINT('Ctrl Pts',(53.3283104451973,11.9999971763164,-6.13292427778441));
#44415=CARTESIAN_POINT('Ctrl Pts',(53.327740031592,11.9999985934556,-6.13237167300935));
#44416=CARTESIAN_POINT('Ctrl Pts',(53.3272835795697,11.999999233682,-6.13192944230248));
#44417=CARTESIAN_POINT('Ctrl Pts',(53.3268952995833,11.9999995977956,-6.13155323347136));
#44418=CARTESIAN_POINT('Ctrl Pts',(53.3265790252902,11.9999998943852,-6.13124679176368));
#44419=CARTESIAN_POINT('Ctrl Pts',(53.3263075195646,12.,-6.13098370645648));
#44420=CARTESIAN_POINT('Ctrl Pts',(53.3260375416529,12.,-6.13072210034901));
#44421=CARTESIAN_POINT('',(53.6630187708265,12.,-5.76570575275302));
#44422=CARTESIAN_POINT('Ctrl Pts',(53.3994258036423,11.9970763379733,-6.20150705299425));
#44423=CARTESIAN_POINT('Ctrl Pts',(53.665710645346,11.9760715488571,-6.45516528751854));
#44424=CARTESIAN_POINT('Ctrl Pts',(54.1171715836631,11.748746829869,-6.8197213266492));
#44425=CARTESIAN_POINT('Ctrl Pts',(54.4602778672668,11.2917992749461,-7.0227986525888));
#44426=CARTESIAN_POINT('Ctrl Pts',(54.5015923607319,11.0939065095575,-7.03987261114144));
#44427=CARTESIAN_POINT('Ctrl Pts',(54.5015923607319,11.,-7.03987261114144));
#44428=CARTESIAN_POINT('Ctrl Pts',(53.6250878309457,11.9970763379733,-5.95707109672624));
#44429=CARTESIAN_POINT('Ctrl Pts',(53.893972841279,11.9760715488571,-6.20791284186137));
#44430=CARTESIAN_POINT('Ctrl Pts',(54.3280790943459,11.748746829869,-6.59126738748239));
#44431=CARTESIAN_POINT('Ctrl Pts',(54.6334138394395,11.2917992749461,-6.83525865116221));
#44432=CARTESIAN_POINT('Ctrl Pts',(54.667728240488,11.0939065095575,-6.8599150740943));
#44433=CARTESIAN_POINT('Ctrl Pts',(54.667728240488,11.,-6.8599150740943));
#44434=CARTESIAN_POINT('Ctrl Pts',(53.8507498582491,11.9970763379733,-5.71263514045823));
#44435=CARTESIAN_POINT('Ctrl Pts',(54.122235037212,11.9760715488571,-5.9606603962042));
#44436=CARTESIAN_POINT('Ctrl Pts',(54.5389866050285,11.748746829869,-6.36281344831557));
#44437=CARTESIAN_POINT('Ctrl Pts',(54.8065498116121,11.2917992749461,-6.64771864973562));
#44438=CARTESIAN_POINT('Ctrl Pts',(54.833864120244,11.0939065095575,-6.67995753704715));
#44439=CARTESIAN_POINT('Ctrl Pts',(54.833864120244,11.,-6.67995753704715));
#44440=CARTESIAN_POINT('Ctrl Pts',(54.0764118855525,11.9970763379733,-5.46819918419023));
#44441=CARTESIAN_POINT('Ctrl Pts',(54.3504972331451,11.9760715488571,-5.71340795054702));
#44442=CARTESIAN_POINT('Ctrl Pts',(54.7498941157113,11.748746829869,-6.13435950914877));
#44443=CARTESIAN_POINT('Ctrl Pts',(54.9796857837848,11.2917992749461,-6.46017864830904));
#44444=CARTESIAN_POINT('Ctrl Pts',(55.,11.0939065095575,-6.5));
#44445=CARTESIAN_POINT('Ctrl Pts',(55.,11.,-6.5));
#44446=CARTESIAN_POINT('Ctrl Pts',(54.0764118855525,11.9970763379733,-5.46819918419023));
#44447=CARTESIAN_POINT('Ctrl Pts',(54.3504972331451,11.9760715488571,-5.71340795054702));
#44448=CARTESIAN_POINT('Ctrl Pts',(54.7498941157113,11.748746829869,-6.13435950914877));
#44449=CARTESIAN_POINT('Ctrl Pts',(54.9796857837848,11.2917992749461,-6.46017864830904));
#44450=CARTESIAN_POINT('Ctrl Pts',(55.,11.0939065095575,-6.5));
#44451=CARTESIAN_POINT('Ctrl Pts',(55.,11.,-6.5));
#44452=CARTESIAN_POINT('Ctrl Pts',(54.5015923607319,11.,-7.03987261114144));
#44453=CARTESIAN_POINT('Ctrl Pts',(54.5015923607319,11.0939065095575,-7.03987261114144));
#44454=CARTESIAN_POINT('Ctrl Pts',(54.4602778672668,11.2917992749461,-7.0227986525888));
#44455=CARTESIAN_POINT('Ctrl Pts',(54.1171715836631,11.748746829869,-6.8197213266492));
#44456=CARTESIAN_POINT('Ctrl Pts',(53.665710645346,11.9760715488571,-6.45516528751854));
#44457=CARTESIAN_POINT('Ctrl Pts',(53.3994258036423,11.9970763379733,-6.20150705299425));
#44458=CARTESIAN_POINT('Origin',(39.3002229812147,11.,-7.25278726518407));
#44459=CARTESIAN_POINT('',(29.9600637960156,12.,-8.));
#44460=CARTESIAN_POINT('Origin',(29.9600637960156,11.,-8.));
#44461=CARTESIAN_POINT('',(39.3002229812147,12.,-7.25278726518407));
#44462=CARTESIAN_POINT('Origin',(23.,8.1,0.));
#44463=CARTESIAN_POINT('',(39.,8.1,-7.));
#44464=CARTESIAN_POINT('',(34.,8.1,6.5));
#44465=CARTESIAN_POINT('',(12.95,8.1,-2.));
#44466=CARTESIAN_POINT('Origin',(16.,8.1,-2.));
#44467=CARTESIAN_POINT('',(-3.05,8.1,3.73517273739943E-16));
#44468=CARTESIAN_POINT('Origin',(0.,8.1,0.));
#44469=CARTESIAN_POINT('Origin',(55.,-12.,-7.));
#44470=CARTESIAN_POINT('',(50.,3.87298334620742,-7.));
#44471=CARTESIAN_POINT('',(50.,3.87298334620742,-7.));
#44472=CARTESIAN_POINT('',(50.,-3.87298334620742,-7.));
#44473=CARTESIAN_POINT('',(50.,-6.,-7.));
#44474=CARTESIAN_POINT('',(50.,-3.87298334620742,-7.));
#44475=CARTESIAN_POINT('Ctrl Pts',(54.0739345923054,-11.9972630926995,7.36867780326845));
#44476=CARTESIAN_POINT('Ctrl Pts',(54.0729086719546,-11.9973391518693,7.36768833576852));
#44477=CARTESIAN_POINT('Ctrl Pts',(54.0688659711553,-11.9976915991107,7.36379269873525));
#44478=CARTESIAN_POINT('Ctrl Pts',(54.0471711411876,-11.9989714998638,7.34303721500929));
#44479=CARTESIAN_POINT('Ctrl Pts',(54.0269258214969,-11.9997129437195,7.32379656765431));
#44480=CARTESIAN_POINT('Ctrl Pts',(54.0051272255687,-12.0000530049878,7.30313001690389));
#44481=CARTESIAN_POINT('Ctrl Pts',(54.0010359532624,-12.,7.29924905261381));
#44482=CARTESIAN_POINT('Ctrl Pts',(54.,-12.,7.29826682694392));
#44483=CARTESIAN_POINT('Ctrl Pts',(53.8388489959598,-11.9972630926995,7.6037633996141));
#44484=CARTESIAN_POINT('Ctrl Pts',(53.8378352265592,-11.9973391518693,7.60276178116386));
#44485=CARTESIAN_POINT('Ctrl Pts',(53.8338827986705,-11.9976915991107,7.59877587122005));
#44486=CARTESIAN_POINT('Ctrl Pts',(53.8124635143653,-11.9989714998638,7.57774484183155));
#44487=CARTESIAN_POINT('Ctrl Pts',(53.7926063578387,-11.9997129437195,7.5581160313125));
#44488=CARTESIAN_POINT('Ctrl Pts',(53.771093178854,-12.0000530049878,7.53716406361864));
#44489=CARTESIAN_POINT('Ctrl Pts',(53.7671069863795,-12.,7.53317801949668));
#44490=CARTESIAN_POINT('Ctrl Pts',(53.7660889423146,-12.,7.53217788462928));
#44491=CARTESIAN_POINT('Ctrl Pts',(53.6037633996141,-11.9972630926995,7.83884899595975));
#44492=CARTESIAN_POINT('Ctrl Pts',(53.6027617811639,-11.9973391518693,7.8378352265592));
#44493=CARTESIAN_POINT('Ctrl Pts',(53.59877587122,-11.9982153918639,7.83387226013102));
#44494=CARTESIAN_POINT('Ctrl Pts',(53.5777448418315,-11.9985200268038,7.81218733844659));
#44495=CARTESIAN_POINT('Ctrl Pts',(53.5581160313125,-12.0001842955338,7.79240311946324));
#44496=CARTESIAN_POINT('Ctrl Pts',(53.5371640636186,-11.999532009425,7.77100498101964));
#44497=CARTESIAN_POINT('Ctrl Pts',(53.5331780194967,-12.,7.76710698637954));
#44498=CARTESIAN_POINT('Ctrl Pts',(53.5321778846293,-12.,7.76608894231464));
#44499=CARTESIAN_POINT('Ctrl Pts',(53.3686778032684,-11.9972630926995,8.0739345923054));
#44500=CARTESIAN_POINT('Ctrl Pts',(53.3676883357685,-11.9973391518693,8.07290867195454));
#44501=CARTESIAN_POINT('Ctrl Pts',(53.3637926987352,-11.9976915991107,8.0688659711553));
#44502=CARTESIAN_POINT('Ctrl Pts',(53.3430372150093,-11.9989714998638,8.04717114118757));
#44503=CARTESIAN_POINT('Ctrl Pts',(53.3237965676543,-11.9997129437195,8.02692582149689));
#44504=CARTESIAN_POINT('Ctrl Pts',(53.3031300169039,-12.0000530049878,8.00512722556869));
#44505=CARTESIAN_POINT('Ctrl Pts',(53.2992490526138,-12.,8.00103595326241));
#44506=CARTESIAN_POINT('Ctrl Pts',(53.2982668269439,-12.,8.));
#44507=CARTESIAN_POINT('',(53.3686778032684,-11.9972630926995,8.0739345923054));
#44508=CARTESIAN_POINT('Ctrl Pts',(53.3686778032684,-11.9972630926995,8.0739345923054));
#44509=CARTESIAN_POINT('Ctrl Pts',(53.6037633996141,-11.9972630926995,7.83884899595975));
#44510=CARTESIAN_POINT('Ctrl Pts',(53.8388489959598,-11.9972630926995,7.6037633996141));
#44511=CARTESIAN_POINT('Ctrl Pts',(54.0739345923054,-11.9972630926995,7.36867780326845));
#44512=CARTESIAN_POINT('Ctrl Pts',(53.3686778032684,-11.9972630926995,8.0739345923054));
#44513=CARTESIAN_POINT('Ctrl Pts',(53.3683611391569,-11.9972874342867,8.07360626201012));
#44514=CARTESIAN_POINT('Ctrl Pts',(53.3680413192552,-11.9973118857529,8.0732746272395));
#44515=CARTESIAN_POINT('Ctrl Pts',(53.3676471644628,-11.9973417925779,8.0728652782713));
#44516=CARTESIAN_POINT('Ctrl Pts',(53.3672333737902,-11.9973731892917,8.07243553648429));
#44517=CARTESIAN_POINT('Ctrl Pts',(53.3667378598292,-11.9974105876503,8.07192035603661));
#44518=CARTESIAN_POINT('Ctrl Pts',(53.3661183826235,-11.9974566676542,8.07127549475271));
#44519=CARTESIAN_POINT('Ctrl Pts',(53.3654580683611,-11.9975057853351,8.07058812304793));
#44520=CARTESIAN_POINT('Ctrl Pts',(53.3646571866552,-11.9975647402856,8.06975369898109));
#44521=CARTESIAN_POINT('Ctrl Pts',(53.3637054463746,-11.9976331424649,8.06876127584374));
#44522=CARTESIAN_POINT('Ctrl Pts',(53.362653023559,-11.997708780762,8.06766386642043));
#44523=CARTESIAN_POINT('Ctrl Pts',(53.3614165408252,-11.9977958975481,8.0663736798044));
#44524=CARTESIAN_POINT('Ctrl Pts',(53.3600254874228,-11.9978903916136,8.06492123169862));
#44525=CARTESIAN_POINT('Ctrl Pts',(53.3582659835748,-11.9980099144669,8.06308407143828));
#44526=CARTESIAN_POINT('Ctrl Pts',(53.3562600906717,-11.9981409874224,8.06098824295537));
#44527=CARTESIAN_POINT('Ctrl Pts',(53.3541260503937,-11.998272326323,8.05875680809654));
#44528=CARTESIAN_POINT('Ctrl Pts',(53.3519223757936,-11.998407950848,8.05645256090358));
#44529=CARTESIAN_POINT('Ctrl Pts',(53.3495866187313,-11.998543466039,8.05400847853294));
#44530=CARTESIAN_POINT('Ctrl Pts',(53.347256780727,-11.9986694592396,8.0515685095969));
#44531=CARTESIAN_POINT('Ctrl Pts',(53.3454689924396,-11.9987661394242,8.04969621294899));
#44532=CARTESIAN_POINT('Ctrl Pts',(53.3436854660617,-11.998857297748,8.04782715956495));
#44533=CARTESIAN_POINT('Ctrl Pts',(53.3419450818544,-11.9989413499516,8.04600194948922));
#44534=CARTESIAN_POINT('Ctrl Pts',(53.3403729432991,-11.9990172766978,8.04435318531431));
#44535=CARTESIAN_POINT('Ctrl Pts',(53.3388364015668,-11.9990874483239,8.04274061126351));
#44536=CARTESIAN_POINT('Ctrl Pts',(53.3373354567718,-11.9991523945683,8.04116421295797));
#44537=CARTESIAN_POINT('Ctrl Pts',(53.3359014880526,-11.9992144427416,8.03965815766076));
#44538=CARTESIAN_POINT('Ctrl Pts',(53.3345003990797,-11.999271755233,8.03818553003495));
#44539=CARTESIAN_POINT('Ctrl Pts',(53.3330989620326,-11.9993259033641,8.0367115631036));
#44540=CARTESIAN_POINT('Ctrl Pts',(53.3316835335098,-11.9993805920919,8.03522288058259));
#44541=CARTESIAN_POINT('Ctrl Pts',(53.3302615515418,-11.9994322838975,8.03372633218491));
#44542=CARTESIAN_POINT('Ctrl Pts',(53.328804648363,-11.9994816923651,8.03219233801592));
#44543=CARTESIAN_POINT('Ctrl Pts',(53.3272371261908,-11.9995348522934,8.03054187152845));
#44544=CARTESIAN_POINT('Ctrl Pts',(53.3256295253259,-11.9995852953059,8.02884842046903));
#44545=CARTESIAN_POINT('Ctrl Pts',(53.3239879980521,-11.999632219018,8.02711875183636));
#44546=CARTESIAN_POINT('Ctrl Pts',(53.3221078268019,-11.9996859644633,8.02513762530408));
#44547=CARTESIAN_POINT('Ctrl Pts',(53.3201836730757,-11.9997349728798,8.02310953786485));
#44548=CARTESIAN_POINT('Ctrl Pts',(53.3182711113751,-11.999777510105,8.02109337071663));
#44549=CARTESIAN_POINT('Ctrl Pts',(53.315658940947,-11.9998356073061,8.01833969631172));
#44550=CARTESIAN_POINT('Ctrl Pts',(53.3130713611079,-11.9998812347755,8.01561139406509));
#44551=CARTESIAN_POINT('Ctrl Pts',(53.3107102640878,-11.9999139058313,8.01312177294044));
#44552=CARTESIAN_POINT('Ctrl Pts',(53.3089394413228,-11.9999384091233,8.01125455709695));
#44553=CARTESIAN_POINT('Ctrl Pts',(53.3072984621054,-11.9999557986327,8.00952417278428));
#44554=CARTESIAN_POINT('Ctrl Pts',(53.3058574649829,-11.9999679622468,8.00800465364294));
#44555=CARTESIAN_POINT('Ctrl Pts',(53.3046394106088,-11.9999782439768,8.006720225723));
#44556=CARTESIAN_POINT('Ctrl Pts',(53.3035646306533,-11.9999848583685,8.00558686693279));
#44557=CARTESIAN_POINT('Ctrl Pts',(53.3026501024977,-11.9999893162497,8.0046224870448));
#44558=CARTESIAN_POINT('Ctrl Pts',(53.3017902315958,-11.9999935077033,8.00371574382527));
#44559=CARTESIAN_POINT('Ctrl Pts',(53.3010724325772,-11.9999958172979,8.00295880824015));
#44560=CARTESIAN_POINT('Ctrl Pts',(53.3004808769946,-11.9999972739225,8.00233498342449));
#44561=CARTESIAN_POINT('Ctrl Pts',(53.2999292531747,-11.9999986322206,8.00175326864076));
#44562=CARTESIAN_POINT('Ctrl Pts',(53.2994875514495,-11.999999249454,8.00128745462601));
#44563=CARTESIAN_POINT('Ctrl Pts',(53.299112508452,-11.9999996022395,8.00089191980187));
#44564=CARTESIAN_POINT('Ctrl Pts',(53.2987993493698,-11.9999998968136,8.00056165014393));
#44565=CARTESIAN_POINT('Ctrl Pts',(53.2985322795654,-12.,8.00027997283885));
#44566=CARTESIAN_POINT('Ctrl Pts',(53.2982668269439,-12.,8.));
#44567=CARTESIAN_POINT('Ctrl Pts',(53.3686778032684,11.9972630926995,8.07393459230539));
#44568=CARTESIAN_POINT('Ctrl Pts',(53.3676883357685,11.9973391518693,8.07290867195453));
#44569=CARTESIAN_POINT('Ctrl Pts',(53.3637926987353,11.9976915991107,8.0688659711553));
#44570=CARTESIAN_POINT('Ctrl Pts',(53.3430372150093,11.9989714998638,8.04717114118756));
#44571=CARTESIAN_POINT('Ctrl Pts',(53.3237965676543,11.9997129437196,8.02692582149689));
#44572=CARTESIAN_POINT('Ctrl Pts',(53.3031300169039,12.0000530049878,8.00512722556869));
#44573=CARTESIAN_POINT('Ctrl Pts',(53.2992490526138,12.,8.00103595326241));
#44574=CARTESIAN_POINT('Ctrl Pts',(53.2982668269439,12.,8.));
#44575=CARTESIAN_POINT('Ctrl Pts',(53.6037633996141,11.9972630926995,7.83884899595974));
#44576=CARTESIAN_POINT('Ctrl Pts',(53.6027617811638,11.9973391518693,7.83783522655919));
#44577=CARTESIAN_POINT('Ctrl Pts',(53.5987758712201,11.9976915991107,7.83388279867049));
#44578=CARTESIAN_POINT('Ctrl Pts',(53.5777448418316,11.9989714998638,7.81246351436529));
#44579=CARTESIAN_POINT('Ctrl Pts',(53.5581160313125,11.9997129437196,7.7926063578387));
#44580=CARTESIAN_POINT('Ctrl Pts',(53.5371640636187,12.0000530049878,7.77109317885394));
#44581=CARTESIAN_POINT('Ctrl Pts',(53.5331780194967,12.,7.76710698637954));
#44582=CARTESIAN_POINT('Ctrl Pts',(53.5321778846293,12.,7.76608894231464));
#44583=CARTESIAN_POINT('Ctrl Pts',(53.8388489959597,11.9972630926995,7.60376339961409));
#44584=CARTESIAN_POINT('Ctrl Pts',(53.8378352265592,11.9973391518693,7.60276178116385));
#44585=CARTESIAN_POINT('Ctrl Pts',(53.833872260131,11.9982153918639,7.59877587122005));
#44586=CARTESIAN_POINT('Ctrl Pts',(53.8121873384466,11.9985200268038,7.57774484183155));
#44587=CARTESIAN_POINT('Ctrl Pts',(53.7924031194632,12.0001842955338,7.55811603131252));
#44588=CARTESIAN_POINT('Ctrl Pts',(53.7710049810197,11.999532009425,7.53716406361864));
#44589=CARTESIAN_POINT('Ctrl Pts',(53.7671069863795,12.,7.53317801949667));
#44590=CARTESIAN_POINT('Ctrl Pts',(53.7660889423146,12.,7.53217788462927));
#44591=CARTESIAN_POINT('Ctrl Pts',(54.0739345923054,11.9972630926995,7.36867780326844));
#44592=CARTESIAN_POINT('Ctrl Pts',(54.0729086719545,11.9973391518693,7.36768833576851));
#44593=CARTESIAN_POINT('Ctrl Pts',(54.0688659711553,11.9976915991107,7.36379269873524));
#44594=CARTESIAN_POINT('Ctrl Pts',(54.0471711411876,11.9989714998638,7.34303721500928));
#44595=CARTESIAN_POINT('Ctrl Pts',(54.0269258214969,11.9997129437196,7.32379656765433));
#44596=CARTESIAN_POINT('Ctrl Pts',(54.0051272255687,12.0000530049878,7.30313001690389));
#44597=CARTESIAN_POINT('Ctrl Pts',(54.0010359532624,12.,7.2992490526138));
#44598=CARTESIAN_POINT('Ctrl Pts',(54.,12.,7.29826682694391));
#44599=CARTESIAN_POINT('',(53.2982668269439,12.,8.));
#44600=CARTESIAN_POINT('',(53.3686778032684,11.9972630926995,8.07393459230539));
#44601=CARTESIAN_POINT('Ctrl Pts',(53.2982668269439,12.,8.));
#44602=CARTESIAN_POINT('Ctrl Pts',(53.2985811322872,12.,8.00033149779709));
#44603=CARTESIAN_POINT('Ctrl Pts',(53.2988985821763,11.9999998632791,8.00066630989117));
#44604=CARTESIAN_POINT('Ctrl Pts',(53.2992901434245,11.9999994175998,8.00107925901207));
#44605=CARTESIAN_POINT('Ctrl Pts',(53.2997012071609,11.9999989497226,8.00151277588685));
#44606=CARTESIAN_POINT('Ctrl Pts',(53.3001937467632,11.9999981461834,8.00203219498426));
#44607=CARTESIAN_POINT('Ctrl Pts',(53.3008098989545,11.9999964035612,8.00268195165242));
#44608=CARTESIAN_POINT('Ctrl Pts',(53.3014666575414,11.9999945460946,8.00337452935848));
#44609=CARTESIAN_POINT('Ctrl Pts',(53.302263581072,11.9999916163369,8.00421489865621));
#44610=CARTESIAN_POINT('Ctrl Pts',(53.3032109845114,11.9999864073118,8.00521394204844));
#44611=CARTESIAN_POINT('Ctrl Pts',(53.3042585528888,11.9999806475585,8.00631861005127));
#44612=CARTESIAN_POINT('Ctrl Pts',(53.3054896985523,11.9999720586087,8.00761685387812));
#44613=CARTESIAN_POINT('Ctrl Pts',(53.3068751339638,11.9999587961682,8.00907777317183));
#44614=CARTESIAN_POINT('Ctrl Pts',(53.3086269933134,11.9999420260395,8.0109250805978));
#44615=CARTESIAN_POINT('Ctrl Pts',(53.3106246425574,11.9999175989922,8.01303154298942));
#44616=CARTESIAN_POINT('Ctrl Pts',(53.3127506011298,11.9998833589397,8.01527313050642));
#44617=CARTESIAN_POINT('Ctrl Pts',(53.3149479827775,11.9998479685685,8.01759002573457));
#44618=CARTESIAN_POINT('Ctrl Pts',(53.3172778862811,11.9998020541947,8.02004647877186));
#44619=CARTESIAN_POINT('Ctrl Pts',(53.3196028144622,11.9997469068523,8.0224971606943));
#44620=CARTESIAN_POINT('Ctrl Pts',(53.3213861058047,11.9997046071464,8.02437690901994));
#44621=CARTESIAN_POINT('Ctrl Pts',(53.3231656968351,11.9996570221597,8.0262524447248));
#44622=CARTESIAN_POINT('Ctrl Pts',(53.3249029587413,11.999605600683,8.02808278980505));
#44623=CARTESIAN_POINT('Ctrl Pts',(53.326472213838,11.9995591520651,8.02973612620502));
#44624=CARTESIAN_POINT('Ctrl Pts',(53.3280065398011,11.9995096475949,8.03135217868033));
#44625=CARTESIAN_POINT('Ctrl Pts',(53.3295060480933,11.999457634203,8.03293079764295));
#44626=CARTESIAN_POINT('Ctrl Pts',(53.3309381134142,11.9994079602031,8.03443841549555));
#44627=CARTESIAN_POINT('Ctrl Pts',(53.3323380371434,11.999356061863,8.03591148724446));
#44628=CARTESIAN_POINT('Ctrl Pts',(53.3337390092771,11.9993009489689,8.03738466784339));
#44629=CARTESIAN_POINT('Ctrl Pts',(53.3351545720245,11.9992452620942,8.03887319108083));
#44630=CARTESIAN_POINT('Ctrl Pts',(53.3365774080489,11.9991860424165,8.04036832959046));
#44631=CARTESIAN_POINT('Ctrl Pts',(53.3380358765603,11.9991218195899,8.04189975679361));
#44632=CARTESIAN_POINT('Ctrl Pts',(53.339605020087,11.9990527232523,8.043547395439));
#44633=CARTESIAN_POINT('Ctrl Pts',(53.3412150611489,11.9989777892668,8.04523667284072));
#44634=CARTESIAN_POINT('Ctrl Pts',(53.3428597205588,11.9988967216938,8.04696104118784));
#44635=CARTESIAN_POINT('Ctrl Pts',(53.3447432666844,11.9988038790588,8.04893587397064));
#44636=CARTESIAN_POINT('Ctrl Pts',(53.3466716908128,11.9987029134811,8.05095617475291));
#44637=CARTESIAN_POINT('Ctrl Pts',(53.3485891250862,11.9985964429042,8.05296361221781));
#44638=CARTESIAN_POINT('Ctrl Pts',(53.3512088491728,11.9984509758397,8.05570630455006));
#44639=CARTESIAN_POINT('Ctrl Pts',(53.3538050841659,11.9982950689302,8.05842184964093));
#44640=CARTESIAN_POINT('Ctrl Pts',(53.3561748403525,11.9981439573354,8.06089860782276));
#44641=CARTESIAN_POINT('Ctrl Pts',(53.3579521574925,11.9980306236394,8.06275617645914));
#44642=CARTESIAN_POINT('Ctrl Pts',(53.3595996241856,11.9979203495849,8.06447687506964));
#44643=CARTESIAN_POINT('Ctrl Pts',(53.3610467017614,11.9978204591454,8.06598735720454));
#44644=CARTESIAN_POINT('Ctrl Pts',(53.3622698769639,11.9977360244816,8.06726412655143));
#44645=CARTESIAN_POINT('Ctrl Pts',(53.3633494900304,11.9976591045262,8.06839030066085));
#44646=CARTESIAN_POINT('Ctrl Pts',(53.3642684226497,11.9975925133009,8.06934823289768));
#44647=CARTESIAN_POINT('Ctrl Pts',(53.3651324109649,11.9975299036608,8.07024888898712));
#44648=CARTESIAN_POINT('Ctrl Pts',(53.3658539549706,11.9974764800598,8.0710004010633));
#44649=CARTESIAN_POINT('Ctrl Pts',(53.3664488792868,11.9974320284378,8.07161947114109));
#44650=CARTESIAN_POINT('Ctrl Pts',(53.3670036310318,11.9973905784344,8.07219673819267));
#44651=CARTESIAN_POINT('Ctrl Pts',(53.3674481384678,11.9973569415985,8.07265869230704));
#44652=CARTESIAN_POINT('Ctrl Pts',(53.3678257711913,11.9973282258331,8.07305073549685));
#44653=CARTESIAN_POINT('Ctrl Pts',(53.3681411633075,11.9973042429379,8.07337816297755));
#44654=CARTESIAN_POINT('Ctrl Pts',(53.3684102955234,11.9972836556963,8.07365722934034));
#44655=CARTESIAN_POINT('Ctrl Pts',(53.3686778032684,11.9972630926995,8.07393459230539));
#44656=CARTESIAN_POINT('',(54.0739345923054,11.9972630926995,7.36867780326844));
#44657=CARTESIAN_POINT('Ctrl Pts',(54.0739345923054,11.9972630926995,7.36867780326844));
#44658=CARTESIAN_POINT('Ctrl Pts',(53.8388489959597,11.9972630926995,7.60376339961409));
#44659=CARTESIAN_POINT('Ctrl Pts',(53.6037633996141,11.9972630926995,7.83884899595974));
#44660=CARTESIAN_POINT('Ctrl Pts',(53.3686778032684,11.9972630926995,8.07393459230539));
#44661=CARTESIAN_POINT('',(54.,12.,7.29826682694391));
#44662=CARTESIAN_POINT('Ctrl Pts',(54.0739345923054,11.9972630926995,7.36867780326844));
#44663=CARTESIAN_POINT('Ctrl Pts',(54.0736062620101,11.9972874342867,7.3683611391569));
#44664=CARTESIAN_POINT('Ctrl Pts',(54.0732746272395,11.9973118857528,7.36804131925523));
#44665=CARTESIAN_POINT('Ctrl Pts',(54.0728652782713,11.9973417925779,7.36764716446279));
#44666=CARTESIAN_POINT('Ctrl Pts',(54.0724355364843,11.9973731892917,7.36723337379024));
#44667=CARTESIAN_POINT('Ctrl Pts',(54.0719203560366,11.9974105876503,7.36673785982923));
#44668=CARTESIAN_POINT('Ctrl Pts',(54.0712754947527,11.9974566676542,7.36611838262348));
#44669=CARTESIAN_POINT('Ctrl Pts',(54.0705881230479,11.9975057853351,7.36545806836115));
#44670=CARTESIAN_POINT('Ctrl Pts',(54.0697536989811,11.9975647402856,7.36465718665516));
#44671=CARTESIAN_POINT('Ctrl Pts',(54.0687612758438,11.9976331424649,7.3637054463746));
#44672=CARTESIAN_POINT('Ctrl Pts',(54.0676638664205,11.997708780762,7.36265302355903));
#44673=CARTESIAN_POINT('Ctrl Pts',(54.0663736798044,11.9977958975481,7.36141654082529));
#44674=CARTESIAN_POINT('Ctrl Pts',(54.0649212316987,11.9978903916136,7.36002548742284));
#44675=CARTESIAN_POINT('Ctrl Pts',(54.0630840714383,11.9980099144669,7.35826598357491));
#44676=CARTESIAN_POINT('Ctrl Pts',(54.0609882429554,11.9981409874224,7.3562600906717));
#44677=CARTESIAN_POINT('Ctrl Pts',(54.0587568080966,11.998272326323,7.35412605039371));
#44678=CARTESIAN_POINT('Ctrl Pts',(54.0564525609036,11.998407950848,7.35192237579359));
#44679=CARTESIAN_POINT('Ctrl Pts',(54.0540084785329,11.998543466039,7.34958661873129));
#44680=CARTESIAN_POINT('Ctrl Pts',(54.0515685095969,11.9986694592396,7.34725678072702));
#44681=CARTESIAN_POINT('Ctrl Pts',(54.049696212949,11.9987661394242,7.34546899243955));
#44682=CARTESIAN_POINT('Ctrl Pts',(54.0478271595649,11.9988572977481,7.34368546606171));
#44683=CARTESIAN_POINT('Ctrl Pts',(54.0460019494891,11.9989413499516,7.34194508185438));
#44684=CARTESIAN_POINT('Ctrl Pts',(54.0443531853142,11.9990172766978,7.34037294329907));
#44685=CARTESIAN_POINT('Ctrl Pts',(54.0427406112634,11.9990874483239,7.33883640156666));
#44686=CARTESIAN_POINT('Ctrl Pts',(54.0411642129578,11.9991523945683,7.33733545677172));
#44687=CARTESIAN_POINT('Ctrl Pts',(54.0396581576594,11.9992144427417,7.33590148805134));
#44688=CARTESIAN_POINT('Ctrl Pts',(54.0381855300325,11.9992717552331,7.33450039907735));
#44689=CARTESIAN_POINT('Ctrl Pts',(54.0367115631,11.9993259033642,7.33309896202914));
#44690=CARTESIAN_POINT('Ctrl Pts',(54.0352228805789,11.999380592092,7.33168353350629));
#44691=CARTESIAN_POINT('Ctrl Pts',(54.0337263321811,11.9994322838977,7.33026155153822));
#44692=CARTESIAN_POINT('Ctrl Pts',(54.0321923380121,11.9994816923653,7.32880464835936));
#44693=CARTESIAN_POINT('Ctrl Pts',(54.0305418715244,11.9995348522935,7.32723712618688));
#44694=CARTESIAN_POINT('Ctrl Pts',(54.0288484204647,11.9995852953061,7.32562952532175));
#44695=CARTESIAN_POINT('Ctrl Pts',(54.0271187518318,11.9996322190181,7.32398799804776));
#44696=CARTESIAN_POINT('Ctrl Pts',(54.0251376252991,11.9996859644635,7.32210782679718));
#44697=CARTESIAN_POINT('Ctrl Pts',(54.0231095378595,11.99973497288,7.32018367307067));
#44698=CARTESIAN_POINT('Ctrl Pts',(54.021093370711,11.9997775101051,7.31827111136975));
#44699=CARTESIAN_POINT('Ctrl Pts',(54.0183396963066,11.9998356073062,7.31565894094208));
#44700=CARTESIAN_POINT('Ctrl Pts',(54.0156113940606,11.9998812347755,7.31307136110358));
#44701=CARTESIAN_POINT('Ctrl Pts',(54.0131217729366,11.9999139058314,7.31071026408421));
#44702=CARTESIAN_POINT('Ctrl Pts',(54.0112545570936,11.9999384091233,7.30893944131968));
#44703=CARTESIAN_POINT('Ctrl Pts',(54.0095241727815,11.9999557986327,7.30729846210273));
#44704=CARTESIAN_POINT('Ctrl Pts',(54.0080046536406,11.9999679622468,7.30585746498073));
#44705=CARTESIAN_POINT('Ctrl Pts',(54.0067202257209,11.9999782439769,7.30463941060684));
#44706=CARTESIAN_POINT('Ctrl Pts',(54.0055868669309,11.9999848583685,7.30356463065154));
#44707=CARTESIAN_POINT('Ctrl Pts',(54.0046224870432,11.9999893162497,7.30265010249617));
#44708=CARTESIAN_POINT('Ctrl Pts',(54.0037157438238,11.9999935077033,7.30179023159441));
#44709=CARTESIAN_POINT('Ctrl Pts',(54.0029588082389,11.9999958172979,7.30107243257607));
#44710=CARTESIAN_POINT('Ctrl Pts',(54.0023349834234,11.9999972739225,7.30048087699363));
#44711=CARTESIAN_POINT('Ctrl Pts',(54.0017532686398,11.9999986322206,7.29992925317381));
#44712=CARTESIAN_POINT('Ctrl Pts',(54.0012874546252,11.999999249454,7.29948755144875));
#44713=CARTESIAN_POINT('Ctrl Pts',(54.0008919198012,11.9999996022395,7.29911250845132));
#44714=CARTESIAN_POINT('Ctrl Pts',(54.0005616501435,11.9999998968136,7.29879934936943));
#44715=CARTESIAN_POINT('Ctrl Pts',(54.0002799728386,12.,7.29853227956515));
#44716=CARTESIAN_POINT('Ctrl Pts',(54.,12.,7.29826682694391));
#44717=CARTESIAN_POINT('',(53.649133413472,12.,7.64913341347195));
#44718=CARTESIAN_POINT('Ctrl Pts',(54.0739345923054,11.9972630926995,7.36867780326844));
#44719=CARTESIAN_POINT('Ctrl Pts',(54.3510337690789,11.9767196525453,7.6359311328699));
#44720=CARTESIAN_POINT('Ctrl Pts',(54.7553166986943,11.7446620906573,8.09873418111303));
#44721=CARTESIAN_POINT('Ctrl Pts',(54.9514928044654,11.3451725484551,8.40875696033662));
#44722=CARTESIAN_POINT('Ctrl Pts',(54.9944234105006,11.1325383755072,8.488654852558));
#44723=CARTESIAN_POINT('Ctrl Pts',(55.,11.0439996496616,8.5));
#44724=CARTESIAN_POINT('Ctrl Pts',(55.,11.,8.5));
#44725=CARTESIAN_POINT('Ctrl Pts',(53.8388489959597,11.9972630926995,7.60376339961409));
#44726=CARTESIAN_POINT('Ctrl Pts',(54.1126662236759,11.9767196525453,7.87429867827289));
#44727=CARTESIAN_POINT('Ctrl Pts',(54.5364558595005,11.7446620906573,8.31759502030676));
#44728=CARTESIAN_POINT('Ctrl Pts',(54.7705808564225,11.3451725484551,8.58966890837954));
#44729=CARTESIAN_POINT('Ctrl Pts',(54.8258338911864,11.1325383755072,8.65724437187221));
#44730=CARTESIAN_POINT('Ctrl Pts',(54.8333333333333,11.0439996496616,8.66666666666667));
#44731=CARTESIAN_POINT('Ctrl Pts',(54.8333333333333,11.,8.66666666666667));
#44732=CARTESIAN_POINT('Ctrl Pts',(53.6037633996141,11.9972630926995,7.83884899595974));
#44733=CARTESIAN_POINT('Ctrl Pts',(53.8742986782729,11.9767196525453,8.11266622367587));
#44734=CARTESIAN_POINT('Ctrl Pts',(54.3175950203068,11.7446620906573,8.5364558595005));
#44735=CARTESIAN_POINT('Ctrl Pts',(54.5896689083795,11.3451725484551,8.77058085642246));
#44736=CARTESIAN_POINT('Ctrl Pts',(54.6572443718722,11.1325383755072,8.82583389118641));
#44737=CARTESIAN_POINT('Ctrl Pts',(54.6666666666667,11.0439996496616,8.83333333333333));
#44738=CARTESIAN_POINT('Ctrl Pts',(54.6666666666667,11.,8.83333333333333));
#44739=CARTESIAN_POINT('Ctrl Pts',(53.3686778032684,11.9972630926995,8.07393459230539));
#44740=CARTESIAN_POINT('Ctrl Pts',(53.6359311328699,11.9767196525453,8.35103376907885));
#44741=CARTESIAN_POINT('Ctrl Pts',(54.098734181113,11.7446620906573,8.75531669869423));
#44742=CARTESIAN_POINT('Ctrl Pts',(54.4087569603366,11.3451725484551,8.95149280446538));
#44743=CARTESIAN_POINT('Ctrl Pts',(54.488654852558,11.1325383755072,8.99442341050062));
#44744=CARTESIAN_POINT('Ctrl Pts',(54.5,11.0439996496616,9.));
#44745=CARTESIAN_POINT('Ctrl Pts',(54.5,11.,9.));
#44746=CARTESIAN_POINT('Ctrl Pts',(53.3686778032684,11.9972630926995,8.07393459230539));
#44747=CARTESIAN_POINT('Ctrl Pts',(53.6359311328699,11.9767196525453,8.35103376907885));
#44748=CARTESIAN_POINT('Ctrl Pts',(54.098734181113,11.7446620906573,8.75531669869423));
#44749=CARTESIAN_POINT('Ctrl Pts',(54.4087569603366,11.3451725484551,8.95149280446538));
#44750=CARTESIAN_POINT('Ctrl Pts',(54.488654852558,11.1325383755072,8.99442341050062));
#44751=CARTESIAN_POINT('Ctrl Pts',(54.5,11.0439996496616,9.));
#44752=CARTESIAN_POINT('Ctrl Pts',(54.5,11.,9.));
#44753=CARTESIAN_POINT('',(54.5,11.,9.));
#44754=CARTESIAN_POINT('Ctrl Pts',(55.,11.,8.5));
#44755=CARTESIAN_POINT('Ctrl Pts',(55.,11.0439996496616,8.5));
#44756=CARTESIAN_POINT('Ctrl Pts',(54.9944234105006,11.1325383755072,8.488654852558));
#44757=CARTESIAN_POINT('Ctrl Pts',(54.9514928044654,11.3451725484551,8.40875696033662));
#44758=CARTESIAN_POINT('Ctrl Pts',(54.7553166986943,11.7446620906573,8.09873418111303));
#44759=CARTESIAN_POINT('Ctrl Pts',(54.3510337690789,11.9767196525453,7.6359311328699));
#44760=CARTESIAN_POINT('Ctrl Pts',(54.0739345923054,11.9972630926995,7.36867780326844));
#44761=CARTESIAN_POINT('Origin',(54.75,8.1,8.75));
#44762=CARTESIAN_POINT('',(54.5,-11.,9.));
#44763=CARTESIAN_POINT('Ctrl Pts',(53.3686778032684,-11.9972630926995,8.0739345923054));
#44764=CARTESIAN_POINT('Ctrl Pts',(53.6359311328699,-11.9767196525453,8.35103376907886));
#44765=CARTESIAN_POINT('Ctrl Pts',(54.098734181113,-11.7446620906573,8.75531669869423));
#44766=CARTESIAN_POINT('Ctrl Pts',(54.4087569603366,-11.3451725484551,8.95149280446538));
#44767=CARTESIAN_POINT('Ctrl Pts',(54.488654852558,-11.1325383755072,8.99442341050062));
#44768=CARTESIAN_POINT('Ctrl Pts',(54.5,-11.0439996496616,9.));
#44769=CARTESIAN_POINT('Ctrl Pts',(54.5,-11.,9.));
#44770=CARTESIAN_POINT('Ctrl Pts',(53.6037633996141,-11.9972630926995,7.83884899595975));
#44771=CARTESIAN_POINT('Ctrl Pts',(53.8742986782729,-11.9767196525453,8.11266622367588));
#44772=CARTESIAN_POINT('Ctrl Pts',(54.3175950203067,-11.7446620906573,8.53645585950049));
#44773=CARTESIAN_POINT('Ctrl Pts',(54.5896689083795,-11.3451725484551,8.77058085642246));
#44774=CARTESIAN_POINT('Ctrl Pts',(54.6572443718722,-11.1325383755072,8.82583389118641));
#44775=CARTESIAN_POINT('Ctrl Pts',(54.6666666666667,-11.0439996496616,8.83333333333333));
#44776=CARTESIAN_POINT('Ctrl Pts',(54.6666666666667,-11.,8.83333333333333));
#44777=CARTESIAN_POINT('Ctrl Pts',(53.8388489959598,-11.9972630926995,7.6037633996141));
#44778=CARTESIAN_POINT('Ctrl Pts',(54.1126662236759,-11.9767196525453,7.87429867827289));
#44779=CARTESIAN_POINT('Ctrl Pts',(54.5364558595005,-11.7446620906573,8.31759502030676));
#44780=CARTESIAN_POINT('Ctrl Pts',(54.7705808564224,-11.3451725484551,8.58966890837954));
#44781=CARTESIAN_POINT('Ctrl Pts',(54.8258338911864,-11.1325383755072,8.6572443718722));
#44782=CARTESIAN_POINT('Ctrl Pts',(54.8333333333333,-11.0439996496616,8.66666666666667));
#44783=CARTESIAN_POINT('Ctrl Pts',(54.8333333333333,-11.,8.66666666666667));
#44784=CARTESIAN_POINT('Ctrl Pts',(54.0739345923054,-11.9972630926995,7.36867780326845));
#44785=CARTESIAN_POINT('Ctrl Pts',(54.3510337690789,-11.9767196525453,7.63593113286991));
#44786=CARTESIAN_POINT('Ctrl Pts',(54.7553166986942,-11.7446620906573,8.09873418111303));
#44787=CARTESIAN_POINT('Ctrl Pts',(54.9514928044654,-11.3451725484552,8.40875696033662));
#44788=CARTESIAN_POINT('Ctrl Pts',(54.9944234105006,-11.1325383755072,8.488654852558));
#44789=CARTESIAN_POINT('Ctrl Pts',(55.,-11.0439996496616,8.5));
#44790=CARTESIAN_POINT('Ctrl Pts',(55.,-11.,8.5));
#44791=CARTESIAN_POINT('Ctrl Pts',(54.5,-11.,9.));
#44792=CARTESIAN_POINT('Ctrl Pts',(54.5,-11.0439996496616,9.));
#44793=CARTESIAN_POINT('Ctrl Pts',(54.488654852558,-11.1325383755072,8.99442341050062));
#44794=CARTESIAN_POINT('Ctrl Pts',(54.4087569603366,-11.3451725484551,8.95149280446538));
#44795=CARTESIAN_POINT('Ctrl Pts',(54.098734181113,-11.7446620906573,8.75531669869423));
#44796=CARTESIAN_POINT('Ctrl Pts',(53.6359311328699,-11.9767196525453,8.35103376907886));
#44797=CARTESIAN_POINT('Ctrl Pts',(53.3686778032684,-11.9972630926995,8.0739345923054));
#44798=CARTESIAN_POINT('Origin',(11.5,-11.,8.));
#44799=CARTESIAN_POINT('Origin',(0.,-11.,8.));
#44800=CARTESIAN_POINT('Origin',(11.5,11.,8.));
#44801=CARTESIAN_POINT('',(7.96639400082368E-16,12.,8.));
#44802=CARTESIAN_POINT('',(11.5,12.,8.));
#44803=CARTESIAN_POINT('Origin',(7.96639400082368E-16,11.,8.));
#44804=CARTESIAN_POINT('Origin',(54.,11.,4.5));
#44805=CARTESIAN_POINT('',(54.,12.,4.5));
#44806=CARTESIAN_POINT('Origin',(26.5,11.,-8.));
#44807=CARTESIAN_POINT('',(0.,12.,-8.));
#44808=CARTESIAN_POINT('Origin',(0.,11.,-8.));
#44809=CARTESIAN_POINT('',(26.5,12.,-8.));
#44810=CARTESIAN_POINT('Origin',(0.,11.,0.));
#44811=CARTESIAN_POINT('Origin',(0.,12.,0.));
#44812=CARTESIAN_POINT('Origin',(23.,12.,0.));
#44813=CARTESIAN_POINT('',(12.95,12.,-2.));
#44814=CARTESIAN_POINT('Origin',(16.,12.,-2.));
#44815=CARTESIAN_POINT('',(-3.05,12.,-3.73517273739943E-16));
#44816=CARTESIAN_POINT('Origin',(0.,12.,0.));
#44817=CARTESIAN_POINT('Origin',(26.8002229812147,-11.,-8.25278726518407));
#44818=CARTESIAN_POINT('',(30.,-11.,-9.));
#44819=CARTESIAN_POINT('Origin',(29.9600637960156,-11.,-8.));
#44820=CARTESIAN_POINT('',(26.8799682034976,-11.,-9.24960254372019));
#44821=CARTESIAN_POINT('Origin',(0.,-11.,0.));
#44822=CARTESIAN_POINT('',(0.,-11.,-9.));
#44823=CARTESIAN_POINT('Origin',(0.,-11.,-8.));
#44824=CARTESIAN_POINT('Origin',(0.,-11.,0.));
#44825=CARTESIAN_POINT('Origin',(11.5,-11.,-8.));
#44826=CARTESIAN_POINT('',(11.5,-11.,-9.));
#44827=CARTESIAN_POINT('Origin',(0.,-8.1,-9.));
#44828=CARTESIAN_POINT('',(30.,-8.1,-9.));
#44829=CARTESIAN_POINT('',(0.,-8.1,-9.));
#44830=CARTESIAN_POINT('Origin',(0.,-8.1,0.));
#44831=CARTESIAN_POINT('Origin',(0.,-12.5,0.));
#44832=CARTESIAN_POINT('',(-3.05,-12.5,3.73517273739943E-16));
#44833=CARTESIAN_POINT('Origin',(0.,-12.5,0.));
#44834=CARTESIAN_POINT('',(-3.05,-12.5,3.73517273739943E-16));
#44835=CARTESIAN_POINT('Origin',(16.,-12.5,-2.));
#44836=CARTESIAN_POINT('',(12.95,-12.5,-2.));
#44837=CARTESIAN_POINT('Origin',(16.,-12.5,-2.));
#44838=CARTESIAN_POINT('',(12.95,-12.5,-2.));
#44839=CARTESIAN_POINT('Origin',(50.,0.,0.));
#44840=CARTESIAN_POINT('',(150.,-9.79717439317883E-16,8.));
#44841=CARTESIAN_POINT('Origin',(150.,0.,0.));
#44842=CARTESIAN_POINT('',(50.,-9.79717439317883E-16,8.));
#44843=CARTESIAN_POINT('Origin',(50.,0.,0.));
#44844=CARTESIAN_POINT('Origin',(150.,0.,79.9999999999995));
#44845=CARTESIAN_POINT('',(180.42851484533,-9.79717439317883E-16,14.7458393333612));
#44846=CARTESIAN_POINT('Origin',(183.809460939256,0.,7.49537703706801));
#44847=CARTESIAN_POINT('Origin',(150.,9.79717439317883E-16,79.9999999999995));
#44848=CARTESIAN_POINT('Origin',(183.809460939256,0.,7.49537703706801));
#44849=CARTESIAN_POINT('Origin',(50.,0.,0.));
#44850=CARTESIAN_POINT('Origin',(45.,-12.,6.5));
#44851=CARTESIAN_POINT('Origin',(30.,-8.1,-9.));
#45208=UNCERTAINTY_MEASURE_WITH_UNIT(LENGTH_MEASURE(0.01),#45237,
'DISTANCE_ACCURACY_VALUE',
'Maximum model space distance between geometric entities at asserted c
onnectivities');
#45214=UNCERTAINTY_MEASURE_WITH_UNIT(LENGTH_MEASURE(0.01),#45237,
'DISTANCE_ACCURACY_VALUE',
'Maximum model space distance between geometric entities at asserted c
onnectivities');
#45230=(
GEOMETRIC_REPRESENTATION_CONTEXT(3)
GLOBAL_UNCERTAINTY_ASSIGNED_CONTEXT((#45208))
GLOBAL_UNIT_ASSIGNED_CONTEXT((#45237,#45239,#45240))
REPRESENTATION_CONTEXT('','3D')
);
#45236=(
GEOMETRIC_REPRESENTATION_CONTEXT(3)
GLOBAL_UNCERTAINTY_ASSIGNED_CONTEXT((#45214))
GLOBAL_UNIT_ASSIGNED_CONTEXT((#45237,#45239,#45240))
REPRESENTATION_CONTEXT('','3D')
);
#45237=(
LENGTH_UNIT()
NAMED_UNIT(*)
SI_UNIT(.MILLI.,.METRE.)
);
#45239=(
NAMED_UNIT(*)
PLANE_ANGLE_UNIT()
SI_UNIT($,.RADIAN.)
);
#45240=(
NAMED_UNIT(*)
SI_UNIT($,.STERADIAN.)
SOLID_ANGLE_UNIT()
);
#45256=SHAPE_DEFINITION_REPRESENTATION(#45277,#45328);
#45277=PRODUCT_DEFINITION_SHAPE('',$,#45350);
#45328=SHAPE_REPRESENTATION('',(#17879),#45230);
#45334=PRODUCT_DEFINITION_CONTEXT('part definition',#45399,'design');
#45350=PRODUCT_DEFINITION('2026-10-25-23-38-22-272','14_Pump_Handle',#45371,
#45334);
#45371=PRODUCT_DEFINITION_FORMATION('',$,#45416);
#45399=APPLICATION_CONTEXT(
'Core Data for Automotive Mechanical Design Process');
#45400=PRODUCT_CONTEXT('part definition',#45399,'mechanical');
#45416=PRODUCT('2026-10-25-23-38-22-272','14_Pump_Handle',$,(#45400));
#45492=COLOUR_RGB('Off White',0.89,0.88,0.83);
#45493=FILL_AREA_STYLE_COLOUR('',#45492);
#45494=FILL_AREA_STYLE('',(#45493));
#45495=SURFACE_STYLE_FILL_AREA(#45494);
#45496=SURFACE_SIDE_STYLE('',(#45495));
#45497=SURFACE_STYLE_USAGE(.BOTH.,#45496);
#45498=PRESENTATION_STYLE_ASSIGNMENT((#45497));
ENDSEC;
END-ISO-10303-21;
